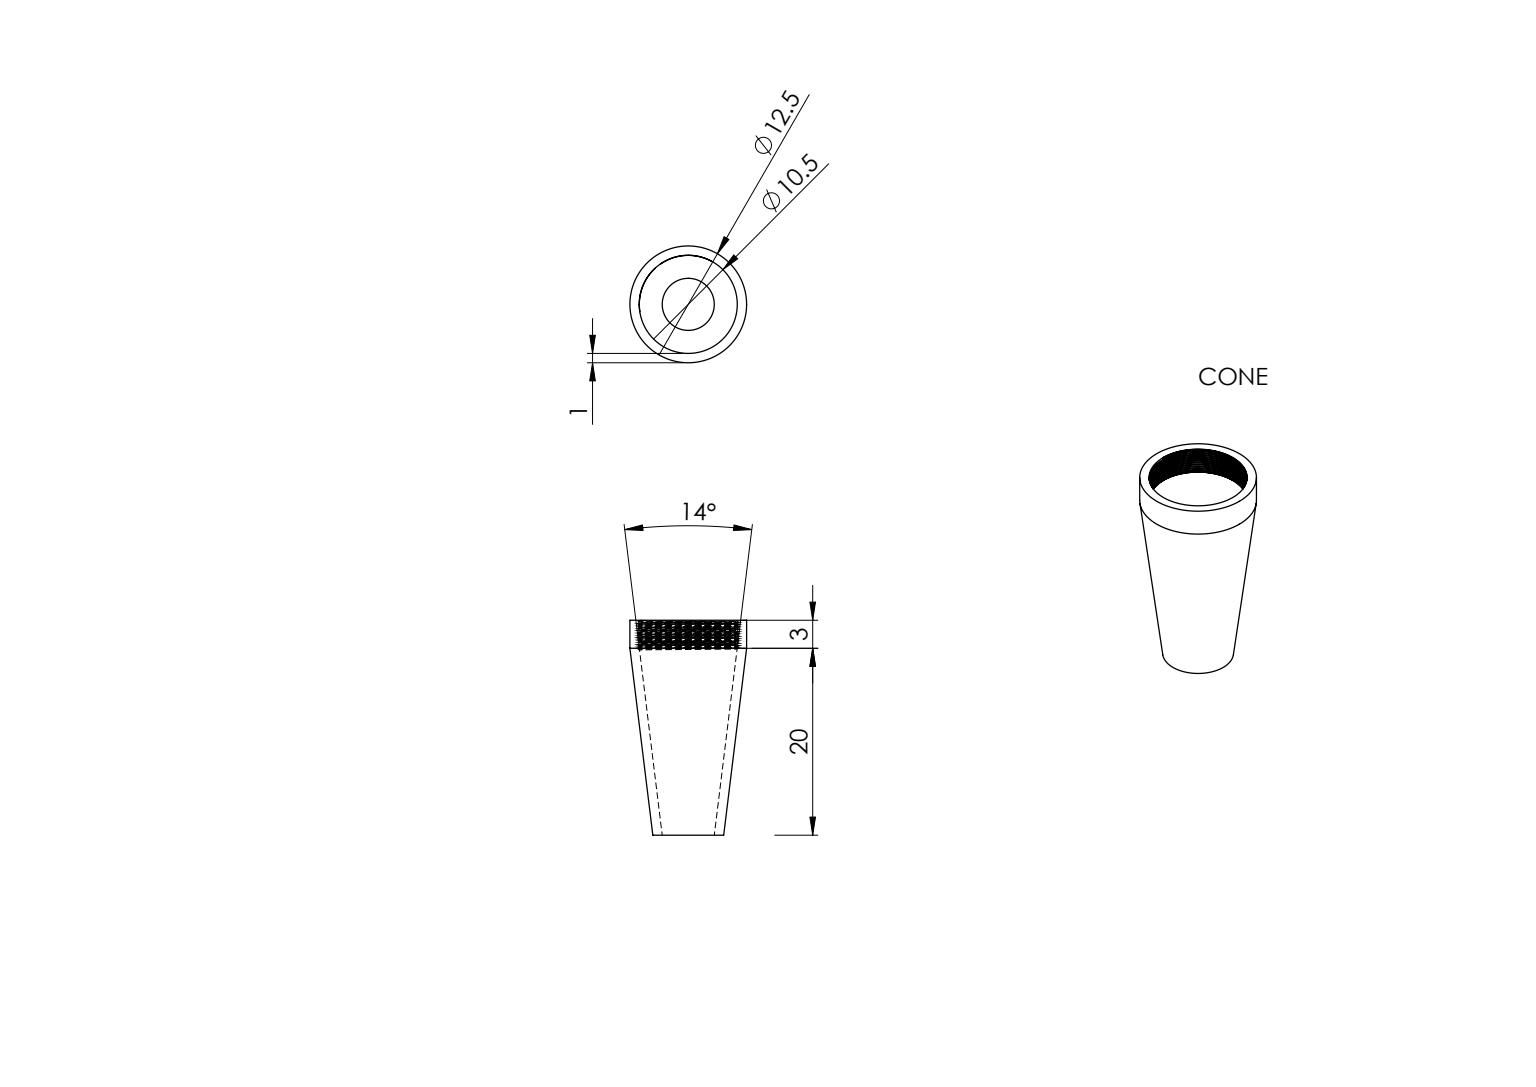
ISO-10303-21;
HEADER;
FILE_DESCRIPTION (('STEP AP214'),
    '1' );
FILE_NAME ('cone.step',
    '2026-10-27T10:49:47',
    ( '' ),
    ( '' ),
    'SwSTEP 2.0',
    'SolidWorks 2026',
    '' );
FILE_SCHEMA (( 'AUTOMOTIVE_DESIGN' ));
ENDSEC;

DATA;
#3=CARTESIAN_POINT ( 'NONE',  ( 1.113604000661152470E-15, -29.93749999999999645, 6.062177826491070398 ) ) ;
#13=CARTESIAN_POINT ( 'NONE',  ( 2.625000000000002220, -29.35416666598386826, 4.546633369868302132 ) ) ;
#14=CARTESIAN_POINT ( 'NONE',  ( 5.249999999999999112, -27.54166666598387181, -3.031088913245536975 ) ) ;
#20=CARTESIAN_POINT ( 'NONE',  ( -5.249999999999997335, -28.91666666598386826, 3.031088913245538308 ) ) ;
#27=VERTEX_POINT ( 'NONE', #2510 ) ;
#29=CARTESIAN_POINT ( 'NONE',  ( 6.429395695523604153E-16, -27.00000000000000000, 5.250000000000000000 ) ) ;
#31=CARTESIAN_POINT ( 'NONE',  ( 2.625000000000002220, -28.91666666666666785, 4.546633369868302132 ) ) ;
#34=CARTESIAN_POINT ( 'NONE',  ( -5.249999999999999112, -28.70833333265053611, -3.031088913245534755 ) ) ;
#38=CARTESIAN_POINT ( 'NONE',  ( 1.406733260263403507, -28.57366454968462577, -5.249999999999994671 ) ) ;
#39=CARTESIAN_POINT ( 'NONE',  ( 5.385316468750000141, -27.73437499965860198, -6.595110575850215044E-16 ) ) ;
#43=APPLICATION_CONTEXT ( 'automotive_design' ) ;
#46=CARTESIAN_POINT ( 'NONE',  ( 5.385316468750000141, -27.45312499965860198, -6.595110575850215044E-16 ) ) ;
#48=ORIENTED_EDGE ( 'NONE', *, *, #6878, .T. ) ;
#49=CARTESIAN_POINT ( 'NONE',  ( -5.385316468750000141, -27.32812499965860198, 0.000000000000000000 ) ) ;
#51=ORIENTED_EDGE ( 'NONE', *, *, #9169, .T. ) ;
#53=CYLINDRICAL_SURFACE ( 'NONE', #3617, 5.250000000000000000 ) ;
#58=CARTESIAN_POINT ( 'NONE',  ( 2.324088772396477476E-15, -27.49999999931720751, -5.250000000000000000 ) ) ;
#60=LINE ( 'NONE', #4208, #5677 ) ;
#63=EDGE_LOOP ( 'NONE', ( #2688, #9138, #7959, #2580 ) ) ;
#64=CARTESIAN_POINT ( 'NONE',  ( 2.161402558328724325E-14, -28.99999999931720751, -5.250000000000000000 ) ) ;
#67=ORIENTED_EDGE ( 'NONE', *, *, #7886, .F. ) ;
#68=DIRECTION ( 'NONE',  ( 0.000000000000000000, -1.000000000000000000, 0.000000000000000000 ) ) ;
#71=EDGE_LOOP ( 'NONE', ( #3557, #48, #247, #244 ) ) ;
#81=CARTESIAN_POINT ( 'NONE',  ( -3.807688866302469071E-16, -28.17187499965860553, -6.218427825808274356 ) ) ;
#85=( BOUNDED_CURVE ( )  B_SPLINE_CURVE ( 2, ( #9078, #8390, #6906, #2534, #530 ),
 .UNSPECIFIED., .F., .F. ) 
 B_SPLINE_CURVE_WITH_KNOTS ( ( 3, 2, 3 ),
 ( 0.9791666666666667407, 0.9861111111111111605, 1.000000000000000000 ),
 .UNSPECIFIED. ) 
 CURVE ( )  GEOMETRIC_REPRESENTATION_ITEM ( )  RATIONAL_B_SPLINE_CURVE ( ( 0.9330127018922192983, 0.9330127018922198534, 1.000000000000000000, 0.8660254037844387076, 1.000000000000000000 ) ) 
 REPRESENTATION_ITEM ( '' )  );
#86=ORIENTED_EDGE ( 'NONE', *, *, #5112, .F. ) ;
#87=CARTESIAN_POINT ( 'NONE',  ( -5.250000000000000000, -29.75000000000000000, 0.000000000000000000 ) ) ;
#97=EDGE_CURVE ( 'NONE', #451, #2823, #2727, .T. ) ;
#98=CARTESIAN_POINT ( 'NONE',  ( 2.161402558328724325E-14, -28.74999999931720751, -5.250000000000000000 ) ) ;
#105=VERTEX_POINT ( 'NONE', #315 ) ;
#106=CARTESIAN_POINT ( 'NONE',  ( -6.972266317189433020E-16, -27.06250000000000000, -5.250000000000000000 ) ) ;
#110=( BOUNDED_CURVE ( )  B_SPLINE_CURVE ( 2, ( #4913, #7058, #9104, #4136, #4827, #6270, #4182, #2042, #682 ),
 .UNSPECIFIED., .F., .T. ) 
 B_SPLINE_CURVE_WITH_KNOTS ( ( 3, 2, 2, 2, 3 ),
 ( 0.3541666666666666852, 0.3611111111111111049, 0.3750000000000000000, 0.3888888888888888951, 0.3958333333333333703 ),
 .UNSPECIFIED. ) 
 CURVE ( )  GEOMETRIC_REPRESENTATION_ITEM ( )  RATIONAL_B_SPLINE_CURVE ( ( 0.9330127018922194093, 0.9330127018922196314, 1.000000000000000000, 0.8660254037844387076, 1.000000000000000000, 0.8660254037844387076, 1.000000000000000000, 0.9330127018922190762, 0.9330127018922194093 ) ) 
 REPRESENTATION_ITEM ( '' )  );
#112=CARTESIAN_POINT ( 'NONE',  ( -2.033577675846918216E-14, -29.68750000000000355, 5.250000000000000888 ) ) ;
#113=CARTESIAN_POINT ( 'NONE',  ( -5.385316468750001029, -27.13020833299193413, -3.109213912904136734 ) ) ;
#119=CARTESIAN_POINT ( 'NONE',  ( -2.033577675846918216E-14, -29.87499999931720396, 5.250000000000000888 ) ) ;
#133=CARTESIAN_POINT ( 'NONE',  ( -5.385316468750000141, -28.82812499965860198, 0.000000000000000000 ) ) ;
#137=CARTESIAN_POINT ( 'NONE',  ( -2.692658234375000514, -27.61979166632526628, -4.663820869356205989 ) ) ;
#144=EDGE_CURVE ( 'NONE', #7348, #2527, #110, .T. ) ;
#160=CARTESIAN_POINT ( 'NONE',  ( 1.975475456537005874E-15, -29.62499999931719685, 5.249999999999999112 ) ) ;
#164=CARTESIAN_POINT ( 'NONE',  ( -2.625000000000000444, -27.97916666598386826, -4.546633369868303021 ) ) ;
#166=( BOUNDED_SURFACE ( )  B_SPLINE_SURFACE ( 1, 2, ( 
 ( #818, #6351, #7897, #2127, #6396, #4313, #4951, #7148, #3203, #6718, #3899, #5281, #6630, #911, #4591, #7235, #8126, #4545, #1608, #8029, #1563, #6587, #3708, #352, #8774, #6533, #1660, #1756, #258, #958, #3109, #3758, #6675, #8725, #7332, #4500, #215, #859, #1053, #7285, #3067, #3804, #3016, #5234, #5886, #5091, #4447, #167, #2357, #7377, #305, #5186, #5841, #6023, #5933, #2404, #8079, #8680, #1707, #1003, #7942, #3849, #2312, #3158, #5976, #8819, #2455, #2263, #5138, #7428, #4404, #7981, #4124, #8269, #545, #7618, #1856, #6123, #7569, #1243, #4085, #4819, #1104, #6920, #1900, #6958, #1989, #4775, #589, #3433, #1946, #3386, #1149, #4683, #3246, #6823, #6218, #8223, #2553, #7663, #8860, #9047, #5420, #6173, #4636, #5373, #7474, #7520, #2500, #399, #2692, #8952, #6772, #3992, #5323, #5519, #8364, #1285, #6070, #8177, #449, #1803, #3295, #6873, #3944, #4728, #1198, #499, #2603, #4041, #8906, #3344, #9000, #2647, #5469, #8315, #2033, #1328, #7703, #4856, #8406, #9093, #5561, #7005, #630 ),
 ( #2737, #6262, #4171, #7436, #8826, #964, #4457, #8135, #1571, #2461, #8086, #5147, #2366, #5099, #918, #7244, #1061, #3117, #868, #5196, #5286, #3811, #4510, #6636, #7294, #1010, #3073, #1667, #8038, #3905, #1713, #4552, #3768, #1618, #175, #6595, #7386, #7989, #8688, #1763, #6728, #3164, #7339, #5940, #4413, #2319, #3718, #225, #359, #6543, #3858, #5894, #3027, #8734, #2272, #4598, #5802, #8640, #5849, #6681, #265, #7949, #8782, #2411, #5242, #311, #5985, #6950, #6995, #2773, #3551, #4115, #2023, #5510, #3463, #579, #8353, #621, #750, #2861, #2724, #703, #4808, #4933, #3423, #5679, #6373, #1978, #4848, #6209, #7694, #4247, #7790, #7127, #5637, #6331, #2063, #2107, #8526, #2680, #9084, #8397, #9038, #6252, #13, #5593, #2816, #7654, #5551, #1277, #7039, #1318, #4891, #1408, #8486, #7743, #4162, #6292, #9128, #1447, #4291, #8437, #9167, #7081, #2155, #664, #1365, #4204, #3508, #4974, #7828, #5912, #4337, #7263, #4428, #797, #1687, #1544, #3641, #4527, #2335, #7172, #5215, #839, #7357 ) ),
 .UNSPECIFIED., .F., .F., .T. ) 
 B_SPLINE_SURFACE_WITH_KNOTS ( ( 2, 2 ),
 ( 3, 2, 2, 2, 2, 2, 2, 2, 2, 2, 2, 2, 2, 2, 2, 2, 2, 2, 2, 2, 2, 2, 2, 2, 2, 2, 2, 2, 2, 2, 2, 2, 2, 2, 2, 2, 2, 2, 2, 2, 2, 2, 2, 2, 2, 2, 2, 2, 2, 2, 2, 2, 2, 2, 2, 2, 2, 2, 2, 2, 2, 2, 2, 2, 2, 2, 2, 2, 2, 2, 2, 2, 3 ),
 ( 0.000000000000000000, 1.000000000000000000 ),
 ( 0.000000000000000000, 0.01388888888888888812, 0.02777777777777777624, 0.04166666666666666435, 0.05555555555555555247, 0.06944444444444444753, 0.08333333333333332871, 0.09722222222222222376, 0.1111111111111111049, 0.1250000000000000000, 0.1388888888888888951, 0.1527777777777777901, 0.1666666666666666574, 0.1805555555555555525, 0.1944444444444444475, 0.2083333333333333426, 0.2222222222222222099, 0.2361111111111111049, 0.2500000000000000000, 0.2638888888888888951, 0.2777777777777777901, 0.2916666666666666852, 0.3055555555555555802, 0.3194444444444444198, 0.3333333333333333148, 0.3472222222222222099, 0.3611111111111111049, 0.3750000000000000000, 0.3888888888888888951, 0.4027777777777777901, 0.4166666666666666852, 0.4305555555555555802, 0.4444444444444444198, 0.4583333333333333148, 0.4722222222222222099, 0.4861111111111111049, 0.5000000000000000000, 0.5138888888888888395, 0.5277777777777777901, 0.5416666666666666297, 0.5555555555555555802, 0.5694444444444444198, 0.5833333333333333703, 0.5972222222222222099, 0.6111111111111111605, 0.6250000000000000000, 0.6388888888888888395, 0.6527777777777777901, 0.6666666666666666297, 0.6805555555555555802, 0.6944444444444444198, 0.7083333333333333703, 0.7222222222222222099, 0.7361111111111111605, 0.7500000000000000000, 0.7638888888888888395, 0.7777777777777777901, 0.7916666666666666297, 0.8055555555555555802, 0.8194444444444444198, 0.8333333333333333703, 0.8472222222222222099, 0.8611111111111111605, 0.8750000000000000000, 0.8888888888888888395, 0.9027777777777777901, 0.9166666666666666297, 0.9305555555555555802, 0.9444444444444444198, 0.9583333333333333703, 0.9722222222222222099, 0.9861111111111111605, 1.000000000000000000 ),
 .UNSPECIFIED. ) 
 GEOMETRIC_REPRESENTATION_ITEM ( )  RATIONAL_B_SPLINE_SURFACE ( (
 ( 1.000000000000000000, 0.8660254037844387076, 1.000000000000000000, 0.8660254037844387076, 1.000000000000000000, 0.8660254037844387076, 1.000000000000000000, 0.8660254037844387076, 1.000000000000000000, 0.8660254037844387076, 1.000000000000000000, 0.8660254037844387076, 1.000000000000000000, 0.8660254037844387076, 1.000000000000000000, 0.8660254037844387076, 1.000000000000000000, 0.8660254037844387076, 1.000000000000000000, 0.8660254037844387076, 1.000000000000000000, 0.8660254037844387076, 1.000000000000000000, 0.8660254037844387076, 1.000000000000000000, 0.8660254037844387076, 1.000000000000000000, 0.8660254037844387076, 1.000000000000000000, 0.8660254037844387076, 1.000000000000000000, 0.8660254037844387076, 1.000000000000000000, 0.8660254037844387076, 1.000000000000000000, 0.8660254037844387076, 1.000000000000000000, 0.8660254037844387076, 1.000000000000000000, 0.8660254037844387076, 1.000000000000000000, 0.8660254037844387076, 1.000000000000000000, 0.8660254037844387076, 1.000000000000000000, 0.8660254037844387076, 1.000000000000000000, 0.8660254037844387076, 1.000000000000000000, 0.8660254037844387076, 1.000000000000000000, 0.8660254037844387076, 1.000000000000000000, 0.8660254037844387076, 1.000000000000000000, 0.8660254037844387076, 1.000000000000000000, 0.8660254037844387076, 1.000000000000000000, 0.8660254037844387076, 1.000000000000000000, 0.8660254037844387076, 1.000000000000000000, 0.8660254037844387076, 1.000000000000000000, 0.8660254037844387076, 1.000000000000000000, 0.8660254037844387076, 1.000000000000000000, 0.8660254037844387076, 1.000000000000000000, 0.8660254037844387076, 1.000000000000000000, 0.8660254037844387076, 1.000000000000000000, 0.8660254037844387076, 1.000000000000000000, 0.8660254037844387076, 1.000000000000000000, 0.8660254037844387076, 1.000000000000000000, 0.8660254037844387076, 1.000000000000000000, 0.8660254037844387076, 1.000000000000000000, 0.8660254037844387076, 1.000000000000000000, 0.8660254037844387076, 1.000000000000000000, 0.8660254037844387076, 1.000000000000000000, 0.8660254037844387076, 1.000000000000000000, 0.8660254037844387076, 1.000000000000000000, 0.8660254037844387076, 1.000000000000000000, 0.8660254037844387076, 1.000000000000000000, 0.8660254037844387076, 1.000000000000000000, 0.8660254037844387076, 1.000000000000000000, 0.8660254037844387076, 1.000000000000000000, 0.8660254037844387076, 1.000000000000000000, 0.8660254037844387076, 1.000000000000000000, 0.8660254037844387076, 1.000000000000000000, 0.8660254037844387076, 1.000000000000000000, 0.8660254037844387076, 1.000000000000000000, 0.8660254037844387076, 1.000000000000000000, 0.8660254037844387076, 1.000000000000000000, 0.8660254037844387076, 1.000000000000000000, 0.8660254037844387076, 1.000000000000000000, 0.8660254037844387076, 1.000000000000000000, 0.8660254037844387076, 1.000000000000000000, 0.8660254037844387076, 1.000000000000000000, 0.8660254037844387076, 1.000000000000000000, 0.8660254037844387076, 1.000000000000000000, 0.8660254037844387076, 1.000000000000000000, 0.8660254037844387076, 1.000000000000000000, 0.8660254037844387076, 1.000000000000000000, 0.8660254037844387076, 1.000000000000000000, 0.8660254037844387076, 1.000000000000000000, 0.8660254037844387076, 1.000000000000000000),
 ( 1.000000000000000000, 0.8660254037844387076, 1.000000000000000000, 0.8660254037844387076, 1.000000000000000000, 0.8660254037844387076, 1.000000000000000000, 0.8660254037844387076, 1.000000000000000000, 0.8660254037844387076, 1.000000000000000000, 0.8660254037844387076, 1.000000000000000000, 0.8660254037844387076, 1.000000000000000000, 0.8660254037844387076, 1.000000000000000000, 0.8660254037844387076, 1.000000000000000000, 0.8660254037844387076, 1.000000000000000000, 0.8660254037844387076, 1.000000000000000000, 0.8660254037844387076, 1.000000000000000000, 0.8660254037844387076, 1.000000000000000000, 0.8660254037844387076, 1.000000000000000000, 0.8660254037844387076, 1.000000000000000000, 0.8660254037844387076, 1.000000000000000000, 0.8660254037844387076, 1.000000000000000000, 0.8660254037844387076, 1.000000000000000000, 0.8660254037844387076, 1.000000000000000000, 0.8660254037844387076, 1.000000000000000000, 0.8660254037844387076, 1.000000000000000000, 0.8660254037844387076, 1.000000000000000000, 0.8660254037844387076, 1.000000000000000000, 0.8660254037844387076, 1.000000000000000000, 0.8660254037844387076, 1.000000000000000000, 0.8660254037844387076, 1.000000000000000000, 0.8660254037844387076, 1.000000000000000000, 0.8660254037844387076, 1.000000000000000000, 0.8660254037844387076, 1.000000000000000000, 0.8660254037844387076, 1.000000000000000000, 0.8660254037844387076, 1.000000000000000000, 0.8660254037844387076, 1.000000000000000000, 0.8660254037844387076, 1.000000000000000000, 0.8660254037844387076, 1.000000000000000000, 0.8660254037844387076, 1.000000000000000000, 0.8660254037844387076, 1.000000000000000000, 0.8660254037844387076, 1.000000000000000000, 0.8660254037844387076, 1.000000000000000000, 0.8660254037844387076, 1.000000000000000000, 0.8660254037844387076, 1.000000000000000000, 0.8660254037844387076, 1.000000000000000000, 0.8660254037844387076, 1.000000000000000000, 0.8660254037844387076, 1.000000000000000000, 0.8660254037844387076, 1.000000000000000000, 0.8660254037844387076, 1.000000000000000000, 0.8660254037844387076, 1.000000000000000000, 0.8660254037844387076, 1.000000000000000000, 0.8660254037844387076, 1.000000000000000000, 0.8660254037844387076, 1.000000000000000000, 0.8660254037844387076, 1.000000000000000000, 0.8660254037844387076, 1.000000000000000000, 0.8660254037844387076, 1.000000000000000000, 0.8660254037844387076, 1.000000000000000000, 0.8660254037844387076, 1.000000000000000000, 0.8660254037844387076, 1.000000000000000000, 0.8660254037844387076, 1.000000000000000000, 0.8660254037844387076, 1.000000000000000000, 0.8660254037844387076, 1.000000000000000000, 0.8660254037844387076, 1.000000000000000000, 0.8660254037844387076, 1.000000000000000000, 0.8660254037844387076, 1.000000000000000000, 0.8660254037844387076, 1.000000000000000000, 0.8660254037844387076, 1.000000000000000000, 0.8660254037844387076, 1.000000000000000000, 0.8660254037844387076, 1.000000000000000000, 0.8660254037844387076, 1.000000000000000000, 0.8660254037844387076, 1.000000000000000000, 0.8660254037844387076, 1.000000000000000000, 0.8660254037844387076, 1.000000000000000000, 0.8660254037844387076, 1.000000000000000000, 0.8660254037844387076, 1.000000000000000000, 0.8660254037844387076, 1.000000000000000000) ) ) 
 REPRESENTATION_ITEM ( '' )  SURFACE ( )  );
#167=CARTESIAN_POINT ( 'NONE',  ( -5.385316468749998364, -28.08854166632526628, 3.109213912904140287 ) ) ;
#170=CARTESIAN_POINT ( 'NONE',  ( 1.142306659890740623E-15, -27.26562499965860553, 6.218427825808274356 ) ) ;
#172=CARTESIAN_POINT ( 'NONE',  ( -5.249999999999997335, -29.41666666598387181, 3.031088913245538308 ) ) ;
#173=EDGE_CURVE ( 'NONE', #105, #7348, #3624, .T. ) ;
#175=CARTESIAN_POINT ( 'NONE',  ( -2.624999999999996891, -27.89583333265053255, 4.546633369868304797 ) ) ;
#180=CARTESIAN_POINT ( 'NONE',  ( 1.142306659890740623E-15, -27.76562499965860198, 6.218427825808274356 ) ) ;
#182=LINE ( 'NONE', #6689, #6964 ) ;
#184=CARTESIAN_POINT ( 'NONE',  ( 2.692658234375002735, -27.24479166632526628, 4.663820869356205101 ) ) ;
#190=AXIS2_PLACEMENT_3D ( 'NONE', #7645, #6857, #8348 ) ;
#194=ADVANCED_FACE ( 'NONE', ( #7672 ), #8416, .F. ) ;
#196=CARTESIAN_POINT ( 'NONE',  ( 7.654042494670957606E-16, -27.00000000000000000, 6.250000000000000000 ) ) ;
#198=CARTESIAN_POINT ( 'NONE',  ( 0.000000000000000000, -50.00000000000000000, 0.000000000000000000 ) ) ;
#206=ADVANCED_FACE ( 'NONE', ( #2793 ), #8063, .F. ) ;
#210=CARTESIAN_POINT ( 'NONE',  ( -5.385316468750001029, -27.88020833299193413, -3.109213912904136734 ) ) ;
#215=CARTESIAN_POINT ( 'NONE',  ( -5.385316468750000141, -27.85937499965860198, 0.000000000000000000 ) ) ;
#221=DIRECTION ( 'NONE',  ( 0.000000000000000000, -1.000000000000000000, 0.000000000000000000 ) ) ;
#225=CARTESIAN_POINT ( 'NONE',  ( -5.249999999999999112, -28.16666666598386826, 3.031088913245538308 ) ) ;
#226=CARTESIAN_POINT ( 'NONE',  ( 1.045839947578414884E-14, -27.81249999999999289, -5.249999999999999112 ) ) ;
#229=CARTESIAN_POINT ( 'NONE',  ( 5.385316468749999252, -27.93229166632526628, -3.109213912904139399 ) ) ;
#231=DIRECTION ( 'NONE',  ( 1.000000000000000000, 0.000000000000000000, -0.000000000000000000 ) ) ;
#233=CARTESIAN_POINT ( 'NONE',  ( 5.385316468750000141, -27.20312499965860198, -6.595110575850215044E-16 ) ) ;
#238=CARTESIAN_POINT ( 'NONE',  ( -5.249999999999999112, -27.47916666666666430, 3.031088913245538308 ) ) ;
#241=DIRECTION ( 'NONE',  ( 0.000000000000000000, -1.000000000000000000, 0.000000000000000000 ) ) ;
#244=ORIENTED_EDGE ( 'NONE', *, *, #7027, .F. ) ;
#247=ORIENTED_EDGE ( 'NONE', *, *, #6707, .T. ) ;
#249=CARTESIAN_POINT ( 'NONE',  ( 0.000000000000000000, -27.00000000000000000, -5.250000000000000000 ) ) ;
#250=CARTESIAN_POINT ( 'NONE',  ( -2.692658234375000514, -28.15104166632526628, -4.663820869356205989 ) ) ;
#252=CARTESIAN_POINT ( 'NONE',  ( 2.625000000000002220, -29.35416666598386826, 4.546633369868302132 ) ) ;
#253=CARTESIAN_POINT ( 'NONE',  ( -2.692658234375000514, -27.90104166632526628, -4.663820869356205989 ) ) ;
#255=CARTESIAN_POINT ( 'NONE',  ( -6.438524027057392246E-16, -29.87813065659485190, 5.257453848358681014 ) ) ;
#258=CARTESIAN_POINT ( 'NONE',  ( 2.692658234374998738, -27.69270833299193768, -4.663820869356206877 ) ) ;
#263=DIRECTION ( 'NONE',  ( 0.000000000000000000, 0.000000000000000000, -1.000000000000000000 ) ) ;
#265=CARTESIAN_POINT ( 'NONE',  ( -5.250000000000000000, -28.43749999931720396, 0.000000000000000000 ) ) ;
#269=DIRECTION ( 'NONE',  ( -1.492469013153037857E-17, 0.9925461516413219831, 0.1218693434051477398 ) ) ;
#271=CARTESIAN_POINT ( 'NONE',  ( -2.692658234374996518, -28.03645833299193413, 4.663820869356208654 ) ) ;
#275=CARTESIAN_POINT ( 'NONE',  ( -5.385316468750001029, -28.34895833299193058, -3.109213912904136734 ) ) ;
#279=VECTOR ( 'NONE', #5592, 1000.000000000000000 ) ;
#281=ORIENTED_EDGE ( 'NONE', *, *, #4233, .T. ) ;
#291=ORIENTED_EDGE ( 'NONE', *, *, #7027, .T. ) ;
#300=CARTESIAN_POINT ( 'NONE',  ( -5.385316468750001029, -27.88020833299193413, -3.109213912904136734 ) ) ;
#301=VERTEX_POINT ( 'NONE', #7582 ) ;
#305=CARTESIAN_POINT ( 'NONE',  ( -2.692658234375000514, -28.15104166632526628, -4.663820869356205989 ) ) ;
#307=ORIENTED_EDGE ( 'NONE', *, *, #1659, .F. ) ;
#310=CARTESIAN_POINT ( 'NONE',  ( 1.975475456537005874E-15, -27.43750000000000000, 5.249999999999999112 ) ) ;
#311=CARTESIAN_POINT ( 'NONE',  ( 5.250000000000000000, -28.54166666598386826, -3.031088913245536531 ) ) ;
#313=EDGE_CURVE ( 'NONE', #7348, #2202, #1209, .T. ) ;
#314=CARTESIAN_POINT ( 'NONE',  ( 0.000000000000000000, -27.00000000000000000, 0.000000000000000000 ) ) ;
#315=CARTESIAN_POINT ( 'NONE',  ( 1.975475456537005874E-15, -28.12499999931720041, 5.249999999999999112 ) ) ;
#317=CARTESIAN_POINT ( 'NONE',  ( 5.385316468750000141, -28.20312499965860198, -6.595110575850215044E-16 ) ) ;
#319=CARTESIAN_POINT ( 'NONE',  ( -2.624999999999996891, -28.45833333333333215, 4.546633369868304797 ) ) ;
#321=CARTESIAN_POINT ( 'NONE',  ( 1.142306659890740623E-15, -28.01562499965860553, 6.218427825808274356 ) ) ;
#323=ORIENTED_EDGE ( 'NONE', *, *, #5988, .F. ) ;
#334=CARTESIAN_POINT ( 'NONE',  ( -5.385316468750000141, -30.09374999965860198, 0.000000000000000000 ) ) ;
#340=VECTOR ( 'NONE', #6184, 1000.000000000000000 ) ;
#342=CARTESIAN_POINT ( 'NONE',  ( -2.692658234374996518, -29.31770833299193413, 4.663820869356208654 ) ) ;
#347=CARTESIAN_POINT ( 'NONE',  ( 5.385316468750001029, -28.75520833299193413, 3.109213912904135846 ) ) ;
#348=EDGE_LOOP ( 'NONE', ( #4332, #2732, #6898, #1040, #4602, #5151, #8448, #421, #7230, #5370, #7405, #1528, #896, #3291, #5973, #7049, #8359, #4121, #7939, #1869, #4062, #7510, #7908, #3823, #5397, #1583, #3967 ) ) ;
#352=CARTESIAN_POINT ( 'NONE',  ( -5.385316468749998364, -27.58854166632526983, 3.109213912904140287 ) ) ;
#354=CARTESIAN_POINT ( 'NONE',  ( -2.692658234374996518, -28.03645833299193413, 4.663820869356208654 ) ) ;
#359=CARTESIAN_POINT ( 'NONE',  ( -5.250000000000000000, -28.18749999931720396, 0.000000000000000000 ) ) ;
#360=CARTESIAN_POINT ( 'NONE',  ( -2.625000000000000444, -28.47916666598386826, -4.546633369868303021 ) ) ;
#365=CARTESIAN_POINT ( 'NONE',  ( 2.692658234374998738, -29.91145833299193413, -4.663820869356206877 ) ) ;
#368=CARTESIAN_POINT ( 'NONE',  ( -5.385316468750000141, -27.09374999965859843, 0.000000000000000000 ) ) ;
#370=CARTESIAN_POINT ( 'NONE',  ( 2.692658234375002735, -27.99479166632526628, 4.663820869356205101 ) ) ;
#374=CARTESIAN_POINT ( 'NONE',  ( 1.406733260263393293, -27.07366454968463287, -5.250000000000000000 ) ) ;
#377=FACE_OUTER_BOUND ( 'NONE', #6458, .T. ) ;
#381=CARTESIAN_POINT ( 'NONE',  ( -6.972266317189433020E-16, -27.56249999999999645, -5.249999999999999112 ) ) ;
#387=( BOUNDED_CURVE ( )  B_SPLINE_CURVE ( 2, ( #1018, #3037, #319, #6552, #8833, #8095, #5950, #3912, #3776 ),
 .UNSPECIFIED., .F., .F. ) 
 B_SPLINE_CURVE_WITH_KNOTS ( ( 3, 2, 2, 2, 3 ),
 ( 0.4791666666666666852, 0.4861111111111111049, 0.5000000000000000000, 0.5138888888888888395, 0.5208333333333333703 ),
 .UNSPECIFIED. ) 
 CURVE ( )  GEOMETRIC_REPRESENTATION_ITEM ( )  RATIONAL_B_SPLINE_CURVE ( ( 0.9330127018922194093, 0.9330127018922196314, 1.000000000000000000, 0.8660254037844387076, 1.000000000000000000, 0.8660254037844387076, 1.000000000000000000, 0.9330127018922187432, 0.9330127018922192983 ) ) 
 REPRESENTATION_ITEM ( '' )  );
#389=FACE_OUTER_BOUND ( 'NONE', #1082, .T. ) ;
#390=CARTESIAN_POINT ( 'NONE',  ( 2.692658234374998738, -29.44270833299193413, -4.663820869356206877 ) ) ;
#394=CARTESIAN_POINT ( 'NONE',  ( 2.692658234375002735, -29.77604166632526983, 4.663820869356205101 ) ) ;
#396=EDGE_LOOP ( 'NONE', ( #8293, #5107, #8604, #2518 ) ) ;
#399=CARTESIAN_POINT ( 'NONE',  ( -5.385316468750001029, -29.38020833299193413, -3.109213912904136734 ) ) ;
#401=CARTESIAN_POINT ( 'NONE',  ( 2.692658234375002735, -28.24479166632526628, 4.663820869356205101 ) ) ;
#410=CARTESIAN_POINT ( 'NONE',  ( -2.692658234375000514, -29.61979166632526983, -4.663820869356205989 ) ) ;
#413=CARTESIAN_POINT ( 'NONE',  ( 2.692658234374998738, -28.41145833299193413, -4.663820869356206877 ) ) ;
#415=ORIENTED_EDGE ( 'NONE', *, *, #2354, .T. ) ;
#421=ORIENTED_EDGE ( 'NONE', *, *, #2572, .T. ) ;
#422=CARTESIAN_POINT ( 'NONE',  ( 5.250000000000000000, -28.35416666666666785, -3.031088913245536531 ) ) ;
#427=LINE ( 'NONE', #7410, #8373 ) ;
#429=CARTESIAN_POINT ( 'NONE',  ( -5.249999999999999112, -29.20833333265053611, -3.031088913245534755 ) ) ;
#435=EDGE_CURVE ( 'NONE', #6343, #8584, #1529, .T. ) ;
#437=ORIENTED_EDGE ( 'NONE', *, *, #2736, .F. ) ;
#439=CARTESIAN_POINT ( 'NONE',  ( 5.385316468750000141, -28.23437499965860198, -6.595110575850215044E-16 ) ) ;
#442=CARTESIAN_POINT ( 'NONE',  ( 2.692658234374998738, -29.44270833299193413, -4.663820869356206877 ) ) ;
#445=ORIENTED_EDGE ( 'NONE', *, *, #3049, .T. ) ;
#449=CARTESIAN_POINT ( 'NONE',  ( -5.385316468750000141, -29.60937499965859843, 0.000000000000000000 ) ) ;
#451=VERTEX_POINT ( 'NONE', #8588 ) ;
#452=CARTESIAN_POINT ( 'NONE',  ( -5.385316468750001029, -28.09895833299192702, -3.109213912904136734 ) ) ;
#457=CARTESIAN_POINT ( 'NONE',  ( 1.975475456537005874E-15, -27.18750000000000000, 5.249999999999999112 ) ) ;
#458=CARTESIAN_POINT ( 'NONE',  ( 1.975475456537005874E-15, -27.43750000000000000, 5.250000000000000000 ) ) ;
#462=CARTESIAN_POINT ( 'NONE',  ( -2.692658234375000514, -29.86979166632526983, -4.663820869356205989 ) ) ;
#465=CARTESIAN_POINT ( 'NONE',  ( 5.385316468750001029, -28.97395833299193413, 3.109213912904135846 ) ) ;
#471=( BOUNDED_CURVE ( )  B_SPLINE_CURVE ( 2, ( #670, #9175, #628, #9136, #1283, #3603, #5600, #2161, #6260 ),
 .UNSPECIFIED., .F., .T. ) 
 B_SPLINE_CURVE_WITH_KNOTS ( ( 3, 2, 2, 2, 3 ),
 ( 0.6875000000000000000, 0.6944444444444444198, 0.7083333333333333703, 0.7222222222222222099, 0.7291666666666667407 ),
 .UNSPECIFIED. ) 
 CURVE ( )  GEOMETRIC_REPRESENTATION_ITEM ( )  RATIONAL_B_SPLINE_CURVE ( ( 0.9330127018922194093, 0.9330127018922194093, 1.000000000000000000, 0.8660254037844387076, 1.000000000000000000, 0.8660254037844387076, 1.000000000000000000, 0.9330127018922187432, 0.9330127018922192983 ) ) 
 REPRESENTATION_ITEM ( '' )  );
#473=( LENGTH_UNIT ( ) NAMED_UNIT ( * ) SI_UNIT ( .MILLI., .METRE. ) );
#474=CARTESIAN_POINT ( 'NONE',  ( 2.625000000000002220, -28.16666666666666785, 4.546633369868302132 ) ) ;
#480=CARTESIAN_POINT ( 'NONE',  ( -2.624999999999996891, -29.14583333265053611, 4.546633369868304797 ) ) ;
#481=ADVANCED_FACE ( 'NONE', ( #820 ), #7102, .F. ) ;
#486=ADVANCED_FACE ( 'NONE', ( #726 ), #5094, .F. ) ;
#487=PLANE ( 'NONE',  #4222 ) ;
#488=CARTESIAN_POINT ( 'NONE',  ( -2.692658234374996518, -28.56770833299193413, 4.663820869356208654 ) ) ;
#489=CARTESIAN_POINT ( 'NONE',  ( -5.385316468750000141, -29.60937499965859843, 0.000000000000000000 ) ) ;
#491=CARTESIAN_POINT ( 'NONE',  ( 2.692658234375002735, -28.77604166632526628, 4.663820869356205101 ) ) ;
#499=CARTESIAN_POINT ( 'NONE',  ( 5.385316468750001029, -29.75520833299193413, 3.109213912904135846 ) ) ;
#503=CARTESIAN_POINT ( 'NONE',  ( -2.692658234374996518, -28.53645833299193413, 4.663820869356208654 ) ) ;
#506=AXIS2_PLACEMENT_3D ( 'NONE', #1402, #9122, #6460 ) ;
#511=DIRECTION ( 'NONE',  ( 0.000000000000000000, 0.000000000000000000, -1.000000000000000000 ) ) ;
#512=CARTESIAN_POINT ( 'NONE',  ( -2.692658234375000514, -29.36979166632526983, -4.663820869356205989 ) ) ;
#516=CARTESIAN_POINT ( 'NONE',  ( -2.692658234374996518, -29.53645833299193413, 4.663820869356208654 ) ) ;
#520=FACE_OUTER_BOUND ( 'NONE', #7413, .T. ) ;
#523=ORIENTED_EDGE ( 'NONE', *, *, #4456, .T. ) ;
#524=CARTESIAN_POINT ( 'NONE',  ( 5.250000000000000888, -28.39583333333333215, 3.031088913245532979 ) ) ;
#530=CARTESIAN_POINT ( 'NONE',  ( -5.250000000000000000, -30.00000000000000000, 0.000000000000000000 ) ) ;
#535=CARTESIAN_POINT ( 'NONE',  ( -5.385316468749998364, -29.08854166632526983, 3.109213912904140287 ) ) ;
#536=CARTESIAN_POINT ( 'NONE',  ( 2.692658234374998738, -29.69270833299193413, -4.663820869356206877 ) ) ;
#538=CARTESIAN_POINT ( 'NONE',  ( 5.385316468750000141, -28.98437499965859843, -6.595110575850215044E-16 ) ) ;
#545=CARTESIAN_POINT ( 'NONE',  ( -2.692658234375000514, -28.65104166632526628, -4.663820869356205989 ) ) ;
#546=EDGE_CURVE ( 'NONE', #27, #4503, #1592, .T. ) ;
#548=CARTESIAN_POINT ( 'NONE',  ( 5.385316468750000141, -28.20312499965860198, -6.595110575850215044E-16 ) ) ;
#551=DIRECTION ( 'NONE',  ( 0.000000000000000000, -1.000000000000000000, 0.000000000000000000 ) ) ;
#558=CARTESIAN_POINT ( 'NONE',  ( -5.385316468750001029, -29.34895833299193413, -3.109213912904136734 ) ) ;
#561=CARTESIAN_POINT ( 'NONE',  ( -2.692658234374996518, -27.31770833299193413, 4.663820869356208654 ) ) ;
#563=DIRECTION ( 'NONE',  ( 0.000000000000000000, 0.000000000000000000, -1.000000000000000000 ) ) ;
#567=CARTESIAN_POINT ( 'NONE',  ( 2.624999999999998668, -28.33333333333333215, -4.546633369868303021 ) ) ;
#570=CARTESIAN_POINT ( 'NONE',  ( 5.250000000000000000, -28.12500000000000000, -6.429395695523604153E-16 ) ) ;
#577=CARTESIAN_POINT ( 'NONE',  ( -5.249999999999997335, -29.22916666666666785, 3.031088913245538308 ) ) ;
#579=CARTESIAN_POINT ( 'NONE',  ( -3.712013335537174572E-16, -28.74999999931720396, -6.062177826491070398 ) ) ;
#580=CARTESIAN_POINT ( 'NONE',  ( -2.692658234375000514, -29.65104166632526983, -4.663820869356205989 ) ) ;
#585=EDGE_LOOP ( 'NONE', ( #8972, #8285, #6547 ) ) ;
#586=AXIS2_PLACEMENT_3D ( 'NONE', #3012, #4443, #8023 ) ;
#589=CARTESIAN_POINT ( 'NONE',  ( 2.692658234374998738, -28.94270833299193413, -4.663820869356206877 ) ) ;
#592=CARTESIAN_POINT ( 'NONE',  ( 1.142306659890740623E-15, -29.01562499965860198, 6.218427825808274356 ) ) ;
#595=CARTESIAN_POINT ( 'NONE',  ( -5.317658234375000070, -27.03906249982929921, 0.000000000000000000 ) ) ;
#597=FACE_OUTER_BOUND ( 'NONE', #7205, .T. ) ;
#599=DIRECTION ( 'NONE',  ( -0.000000000000000000, 1.000000000000000000, -0.000000000000000000 ) ) ;
#601=CARTESIAN_POINT ( 'NONE',  ( -2.625000000000000444, -28.72916666598386826, -4.546633369868303021 ) ) ;
#604=CARTESIAN_POINT ( 'NONE',  ( -3.807688866302469071E-16, -29.39062499965860198, -6.218427825808274356 ) ) ;
#607=CIRCLE ( 'NONE', #1956, 2.786798956483056422 ) ;
#610=VERTEX_POINT ( 'NONE', #1167 ) ;
#611=CARTESIAN_POINT ( 'NONE',  ( -3.712013335537174572E-16, -27.81250000000000000, -6.062177826491070398 ) ) ;
#621=CARTESIAN_POINT ( 'NONE',  ( 5.250000000000000000, -28.79166666598386826, -3.031088913245536531 ) ) ;
#628=CARTESIAN_POINT ( 'NONE',  ( 2.624999999999998668, -29.08333333333333215, -4.546633369868303021 ) ) ;
#630=CARTESIAN_POINT ( 'NONE',  ( -5.385316468750000141, -30.10937499965859843, 0.000000000000000000 ) ) ;
#632=CARTESIAN_POINT ( 'NONE',  ( 5.385316468749999252, -29.43229166632526983, -3.109213912904138954 ) ) ;
#635=CARTESIAN_POINT ( 'NONE',  ( 1.975475456537005874E-15, -28.68749999999999645, 5.249999999999999112 ) ) ;
#644=CARTESIAN_POINT ( 'NONE',  ( 5.385316468750000141, -29.95312499965859843, -6.595110575850215044E-16 ) ) ;
#645=EDGE_CURVE ( 'NONE', #5282, #1598, #1067, .T. ) ;
#648=LINE ( 'NONE', #6317, #9109 ) ;
#653=ORIENTED_EDGE ( 'NONE', *, *, #4489, .T. ) ;
#655=CARTESIAN_POINT ( 'NONE',  ( 5.250000000000000000, -29.37500000000000000, -6.429395695523604153E-16 ) ) ;
#660=CARTESIAN_POINT ( 'NONE',  ( 2.161402558328724325E-14, -29.31250000000000000, -5.250000000000000000 ) ) ;
#663=CARTESIAN_POINT ( 'NONE',  ( -5.250000000000000000, -29.25000000000000000, 0.000000000000000000 ) ) ;
#664=CARTESIAN_POINT ( 'NONE',  ( 5.250000000000000000, -29.79166666598387181, -3.031088913245536531 ) ) ;
#665=CARTESIAN_POINT ( 'NONE',  ( 0.000000000000000000, -27.00000000000000000, -5.250000000000000000 ) ) ;
#670=CARTESIAN_POINT ( 'NONE',  ( -6.972266317189433020E-16, -29.06249999999999645, -5.250000000000000000 ) ) ;
#674=CARTESIAN_POINT ( 'NONE',  ( 5.385316468750001029, -29.22395833299193413, 3.109213912904134958 ) ) ;
#679=FACE_OUTER_BOUND ( 'NONE', #5811, .T. ) ;
#682=CARTESIAN_POINT ( 'NONE',  ( -9.180150650966086169E-15, -28.37499999931720041, 5.250000000000000000 ) ) ;
#685=( BOUNDED_CURVE ( )  B_SPLINE_CURVE ( 2, ( #2269, #6592, #5982, #172, #7986, #7947, #4410, #865, #3715 ),
 .UNSPECIFIED., .F., .F. ) 
 B_SPLINE_CURVE_WITH_KNOTS ( ( 3, 2, 2, 2, 3 ),
 ( 0.7291666666666667407, 0.7361111111111111605, 0.7500000000000000000, 0.7638888888888888395, 0.7708333333333333703 ),
 .UNSPECIFIED. ) 
 CURVE ( )  GEOMETRIC_REPRESENTATION_ITEM ( )  RATIONAL_B_SPLINE_CURVE ( ( 0.9330127018922192983, 0.9330127018922198534, 1.000000000000000000, 0.8660254037844387076, 1.000000000000000000, 0.8660254037844387076, 1.000000000000000000, 0.9330127018922187432, 0.9330127018922192983 ) ) 
 REPRESENTATION_ITEM ( '' )  );
#687=CARTESIAN_POINT ( 'NONE',  ( -2.692658234375000514, -29.61979166632526983, -4.663820869356205989 ) ) ;
#694=CARTESIAN_POINT ( 'NONE',  ( 5.250000000000000888, -29.39583333333332860, 3.031088913245532979 ) ) ;
#703=CARTESIAN_POINT ( 'NONE',  ( 1.113604000661152470E-15, -28.87499999931720396, 6.062177826491070398 ) ) ;
#706=CARTESIAN_POINT ( 'NONE',  ( -2.692658234374996518, -30.06770833299193413, 4.663820869356208654 ) ) ;
#713=ADVANCED_FACE ( 'NONE', ( #520 ), #7635, .F. ) ;
#715=ORIENTED_EDGE ( 'NONE', *, *, #4351, .T. ) ;
#716=CARTESIAN_POINT ( 'NONE',  ( -3.807688866302469071E-16, -29.89062499965859843, -6.218427825808274356 ) ) ;
#722=DIRECTION ( 'NONE',  ( 0.000000000000000000, 0.000000000000000000, -1.000000000000000000 ) ) ;
#726=FACE_OUTER_BOUND ( 'NONE', #1560, .T. ) ;
#730=CARTESIAN_POINT ( 'NONE',  ( -5.385316468750001029, -28.38020833299193058, -3.109213912904136734 ) ) ;
#737=CARTESIAN_POINT ( 'NONE',  ( -5.250000000000000000, -29.25000000000000000, 0.000000000000000000 ) ) ;
#739=CARTESIAN_POINT ( 'NONE',  ( -1.406733260263393070, -27.30133545031536357, -5.250000000000000888 ) ) ;
#743=EDGE_LOOP ( 'NONE', ( #7927, #7894 ) ) ;
#750=CARTESIAN_POINT ( 'NONE',  ( 5.250000000000000000, -28.81249999931720396, -6.429395695523604153E-16 ) ) ;
#751=CARTESIAN_POINT ( 'NONE',  ( 5.250000000000000000, -27.56249999931720396, -6.429395695523604153E-16 ) ) ;
#757=EDGE_LOOP ( 'NONE', ( #8210, #7399, #8601, #6496 ) ) ;
#759=CARTESIAN_POINT ( 'NONE',  ( -1.406733260263394625, -27.55133545031536713, -5.250000000000000000 ) ) ;
#761=EDGE_CURVE ( 'NONE', #7091, #2823, #648, .T. ) ;
#764=ORIENTED_EDGE ( 'NONE', *, *, #4966, .T. ) ;
#765=CARTESIAN_POINT ( 'NONE',  ( 5.385316468750000141, -29.70312499965859843, -6.595110575850215044E-16 ) ) ;
#767=CARTESIAN_POINT ( 'NONE',  ( 6.429395695523604153E-16, -27.00000000000000000, 5.250000000000000000 ) ) ;
#770=CARTESIAN_POINT ( 'NONE',  ( -6.972266317189433020E-16, -29.06249999999999645, -5.250000000000000000 ) ) ;
#771=CARTESIAN_POINT ( 'NONE',  ( 6.429395695523604153E-16, -27.00000000000000000, 5.250000000000000000 ) ) ;
#772=CARTESIAN_POINT ( 'NONE',  ( 5.250000000000000888, -27.33333333265053611, 3.031088913245533423 ) ) ;
#778=CARTESIAN_POINT ( 'NONE',  ( -2.692658234375000514, -27.65104166632526628, -4.663820869356205989 ) ) ;
#785=AXIS2_PLACEMENT_3D ( 'NONE', #1263, #6935, #563 ) ;
#786=CARTESIAN_POINT ( 'NONE',  ( 2.692658234375002735, -27.49479166632526628, 4.663820869356205101 ) ) ;
#788=ORIENTED_EDGE ( 'NONE', *, *, #7385, .F. ) ;
#797=CARTESIAN_POINT ( 'NONE',  ( -3.712013335537174572E-16, -29.99999999931720041, -6.062177826491070398 ) ) ;
#800=CARTESIAN_POINT ( 'NONE',  ( -5.250000000000000000, -27.75000000000000000, 0.000000000000000000 ) ) ;
#807=EDGE_LOOP ( 'NONE', ( #1458, #4944, #5003, #5759 ) ) ;
#809=CARTESIAN_POINT ( 'NONE',  ( 5.249999999999999112, -29.60416666666666785, -3.031088913245536975 ) ) ;
#812=CARTESIAN_POINT ( 'NONE',  ( 5.250000000000000888, -29.33333333265053611, 3.031088913245533423 ) ) ;
#814=EDGE_CURVE ( 'NONE', #4395, #3226, #6461, .T. ) ;
#818=CARTESIAN_POINT ( 'NONE',  ( -5.385316468750000141, -27.10937499965860198, 0.000000000000000000 ) ) ;
#820=FACE_OUTER_BOUND ( 'NONE', #3345, .T. ) ;
#821=CARTESIAN_POINT ( 'NONE',  ( 2.692658234374998738, -27.16145833299193413, -4.663820869356206877 ) ) ;
#823=CARTESIAN_POINT ( 'NONE',  ( 0.000000000000000000, -27.00000000000000000, 0.000000000000000000 ) ) ;
#824=CARTESIAN_POINT ( 'NONE',  ( 2.692658234375002735, -28.52604166632526628, 4.663820869356205101 ) ) ;
#829=CARTESIAN_POINT ( 'NONE',  ( 2.624999999999998668, -29.02083333265053611, -4.546633369868303021 ) ) ;
#830=EDGE_LOOP ( 'NONE', ( #2328, #67 ) ) ;
#831=CARTESIAN_POINT ( 'NONE',  ( 2.625000000000002220, -29.66666666666666785, 4.546633369868302132 ) ) ;
#839=CARTESIAN_POINT ( 'NONE',  ( -5.249999999999999112, -30.16666666598386470, 3.031088913245538308 ) ) ;
#841=LINE ( 'NONE', #941, #8467 ) ;
#842=CARTESIAN_POINT ( 'NONE',  ( -2.624999999999996891, -28.20833333333333215, 4.546633369868304797 ) ) ;
#843=CARTESIAN_POINT ( 'NONE',  ( 0.000000000000000000, -29.87813065659485190, -5.257453848358681014 ) ) ;
#846=CARTESIAN_POINT ( 'NONE',  ( 5.250000000000000888, -27.14583333333332860, 3.031088913245533423 ) ) ;
#851=EDGE_CURVE ( 'NONE', #8796, #3220, #8383, .T. ) ;
#854=CARTESIAN_POINT ( 'NONE',  ( 5.385316468749999252, -27.21354166632526628, -3.109213912904138954 ) ) ;
#857=CARTESIAN_POINT ( 'NONE',  ( 5.249999999999999112, -29.85416666666666785, -3.031088913245536975 ) ) ;
#859=CARTESIAN_POINT ( 'NONE',  ( -5.385316468750001029, -27.88020833299193413, -3.109213912904136734 ) ) ;
#860=UNCERTAINTY_MEASURE_WITH_UNIT (LENGTH_MEASURE( 1.000000000000000082E-05 ), #473, 'distance_accuracy_value', 'NONE');
#863=CARTESIAN_POINT ( 'NONE',  ( 5.385316468749999252, -27.18229166632526628, -3.109213912904138954 ) ) ;
#865=CARTESIAN_POINT ( 'NONE',  ( -1.406733260263384411, -29.48883544963257464, -5.250000000000006217 ) ) ;
#868=CARTESIAN_POINT ( 'NONE',  ( 5.250000000000000000, -27.56249999931720396, -6.429395695523604153E-16 ) ) ;
#869=CARTESIAN_POINT ( 'NONE',  ( 5.250000000000000888, -27.64583333333333570, 3.031088913245533423 ) ) ;
#876=CARTESIAN_POINT ( 'NONE',  ( 2.692658234374998738, -27.91145833299193413, -4.663820869356206877 ) ) ;
#888=AXIS2_PLACEMENT_3D ( 'NONE', #4026, #9081, #6861 ) ;
#889=CARTESIAN_POINT ( 'NONE',  ( -2.625000000000000444, -27.04166666666666430, -4.546633369868303021 ) ) ;
#896=ORIENTED_EDGE ( 'NONE', *, *, #7076, .T. ) ;
#904=CARTESIAN_POINT ( 'NONE',  ( -5.385316468750000141, -27.85937499965860198, 0.000000000000000000 ) ) ;
#911=CARTESIAN_POINT ( 'NONE',  ( -5.385316468750001029, -27.38020833299193768, -3.109213912904136734 ) ) ;
#913=DIRECTION ( 'NONE',  ( 0.000000000000000000, 0.000000000000000000, -1.000000000000000000 ) ) ;
#914=CARTESIAN_POINT ( 'NONE',  ( -5.385316468749998364, -27.55729166632526628, 3.109213912904140287 ) ) ;
#916=CARTESIAN_POINT ( 'NONE',  ( 1.975475456537005874E-15, -27.37499999931720041, 5.250000000000000000 ) ) ;
#918=CARTESIAN_POINT ( 'NONE',  ( -2.625000000000000444, -27.47916666598386826, -4.546633369868303021 ) ) ;
#923=CARTESIAN_POINT ( 'NONE',  ( -2.692658234375000514, -28.11979166632526628, -4.663820869356205989 ) ) ;
#924=EDGE_CURVE ( 'NONE', #8014, #8128, #5623, .T. ) ;
#927=ORIENTED_EDGE ( 'NONE', *, *, #5310, .F. ) ;
#928=CARTESIAN_POINT ( 'NONE',  ( -2.624999999999996891, -27.20833333333333570, 4.546633369868304797 ) ) ;
#938=CARTESIAN_POINT ( 'NONE',  ( 5.250000000000000888, -27.14583333333333570, 3.031088913245532979 ) ) ;
#941=CARTESIAN_POINT ( 'NONE',  ( 6.429395695523604153E-16, -27.00000000000000000, 5.250000000000000000 ) ) ;
#942=CARTESIAN_POINT ( 'NONE',  ( -5.250000000000000000, -28.25000000000000000, 0.000000000000000000 ) ) ;
#946=VERTEX_POINT ( 'NONE', #226 ) ;
#949=ORIENTED_EDGE ( 'NONE', *, *, #4125, .F. ) ;
#951=CARTESIAN_POINT ( 'NONE',  ( -5.385316468750001029, -27.38020833299193058, -3.109213912904136734 ) ) ;
#958=CARTESIAN_POINT ( 'NONE',  ( 5.385316468749999252, -27.71354166632526272, -3.109213912904139399 ) ) ;
#961=CARTESIAN_POINT ( 'NONE',  ( -2.692658234374996518, -27.53645833299193413, 4.663820869356208654 ) ) ;
#964=CARTESIAN_POINT ( 'NONE',  ( 5.250000000000000000, -27.29166666598386826, -3.031088913245536531 ) ) ;
#965=CARTESIAN_POINT ( 'NONE',  ( 1.975475456537005874E-15, -27.62499999931720041, 5.250000000000000000 ) ) ;
#967=CARTESIAN_POINT ( 'NONE',  ( -2.033577675846918216E-14, -29.87499999931720396, 5.250000000000000888 ) ) ;
#970=CARTESIAN_POINT ( 'NONE',  ( 2.692658234375002735, -28.24479166632526628, 4.663820869356205101 ) ) ;
#971=ADVANCED_FACE ( 'NONE', ( #8322 ), #8915, .F. ) ;
#975=CARTESIAN_POINT ( 'NONE',  ( 2.692658234374998738, -28.91145833299193413, -4.663820869356206877 ) ) ;
#982=( BOUNDED_CURVE ( )  B_SPLINE_CURVE ( 2, ( #6188, #1260, #4831, #7587, #2619, #8921, #5436, #6273, #2006 ),
 .UNSPECIFIED., .F., .F. ) 
 B_SPLINE_CURVE_WITH_KNOTS ( ( 3, 2, 2, 2, 3 ),
 ( 0.3125000000000000000, 0.3194444444444444198, 0.3333333333333333148, 0.3472222222222222099, 0.3541666666666666852 ),
 .UNSPECIFIED. ) 
 CURVE ( )  GEOMETRIC_REPRESENTATION_ITEM ( )  RATIONAL_B_SPLINE_CURVE ( ( 0.9330127018922194093, 0.9330127018922194093, 1.000000000000000000, 0.8660254037844387076, 1.000000000000000000, 0.8660254037844387076, 1.000000000000000000, 0.9330127018922190762, 0.9330127018922194093 ) ) 
 REPRESENTATION_ITEM ( '' )  );
#985=CARTESIAN_POINT ( 'NONE',  ( -1.406733260263394625, -28.30133545031536713, -5.250000000000000000 ) ) ;
#994=CARTESIAN_POINT ( 'NONE',  ( 2.692658234374998738, -27.69270833299193768, -4.663820869356206877 ) ) ;
#996=UNCERTAINTY_MEASURE_WITH_UNIT (LENGTH_MEASURE( 1.000000000000000082E-05 ), #5266, 'distance_accuracy_value', 'NONE');
#998=CARTESIAN_POINT ( 'NONE',  ( -3.807688866302469071E-16, -27.92187499965860198, -6.218427825808274356 ) ) ;
#999=ORIENTED_EDGE ( 'NONE', *, *, #4125, .T. ) ;
#1003=CARTESIAN_POINT ( 'NONE',  ( -5.385316468749998364, -28.33854166632526628, 3.109213912904140287 ) ) ;
#1005=EDGE_LOOP ( 'NONE', ( #5857, #7682, #7845, #1554 ) ) ;
#1010=CARTESIAN_POINT ( 'NONE',  ( -5.250000000000000000, -27.70833333265053611, -3.031088913245534755 ) ) ;
#1012=DIRECTION ( 'NONE',  ( 0.000000000000000000, 0.000000000000000000, -1.000000000000000000 ) ) ;
#1013=CARTESIAN_POINT ( 'NONE',  ( 1.406733260263385521, -29.11383544963257464, 5.250000000000006217 ) ) ;
#1016=CARTESIAN_POINT ( 'NONE',  ( -5.385316468749998364, -28.05729166632526983, 3.109213912904140287 ) ) ;
#1018=CARTESIAN_POINT ( 'NONE',  ( -9.180150650966086169E-15, -28.43750000000000000, 5.250000000000000000 ) ) ;
#1020=CARTESIAN_POINT ( 'NONE',  ( -5.385316468750000141, -27.82812499965860198, 0.000000000000000000 ) ) ;
#1026=ORIENTED_EDGE ( 'NONE', *, *, #3740, .T. ) ;
#1028=CARTESIAN_POINT ( 'NONE',  ( 5.250000000000000888, -27.39583333333333215, 3.031088913245532979 ) ) ;
#1035=ORIENTED_EDGE ( 'NONE', *, *, #6208, .T. ) ;
#1040=ORIENTED_EDGE ( 'NONE', *, *, #7385, .T. ) ;
#1044=CARTESIAN_POINT ( 'NONE',  ( -5.385316468749998364, -28.33854166632526628, 3.109213912904140287 ) ) ;
#1047=CARTESIAN_POINT ( 'NONE',  ( -5.385316468749998364, -28.33854166632526628, 3.109213912904140287 ) ) ;
#1053=CARTESIAN_POINT ( 'NONE',  ( -2.692658234375000514, -27.90104166632526628, -4.663820869356205989 ) ) ;
#1058=CARTESIAN_POINT ( 'NONE',  ( -5.385316468750000141, -27.82812499965860198, 0.000000000000000000 ) ) ;
#1061=CARTESIAN_POINT ( 'NONE',  ( 2.624999999999998668, -27.52083333265053611, -4.546633369868303021 ) ) ;
#1067=( BOUNDED_CURVE ( )  B_SPLINE_CURVE ( 2, ( #2665, #1920, #5537, #4010, #2757, #7722, #6844, #3964, #1877, #5392, #1965 ),
 .UNSPECIFIED., .F., .F. ) 
 B_SPLINE_CURVE_WITH_KNOTS ( ( 3, 2, 2, 2, 2, 3 ),
 ( 0.9375000002123526910, 0.9444444444444444198, 0.9583333333333333703, 0.9722222222222222099, 0.9861111111111111605, 1.000000000000000000 ),
 .UNSPECIFIED. ) 
 CURVE ( )  GEOMETRIC_REPRESENTATION_ITEM ( )  RATIONAL_B_SPLINE_CURVE ( ( 0.9330127018922194093, 0.9330127039406097555, 1.000000000000000000, 0.8660254037844387076, 1.000000000000000000, 0.8660254037844387076, 1.000000000000000000, 0.8660254037844387076, 1.000000000000000000, 0.8660254037844387076, 1.000000000000000000 ) ) 
 REPRESENTATION_ITEM ( '' )  );
#1068=CARTESIAN_POINT ( 'NONE',  ( -2.692658234375000514, -28.36979166632526628, -4.663820869356205989 ) ) ;
#1072=CARTESIAN_POINT ( 'NONE',  ( -3.807688866302469071E-16, -27.89062499965860198, -6.218427825808274356 ) ) ;
#1074=VERTEX_POINT ( 'NONE', #457 ) ;
#1079=ORIENTED_EDGE ( 'NONE', *, *, #8052, .F. ) ;
#1081=CARTESIAN_POINT ( 'NONE',  ( -3.712013335537174572E-16, -27.06250000000000000, -6.062177826491070398 ) ) ;
#1082=EDGE_LOOP ( 'NONE', ( #8172, #4837 ) ) ;
#1086=DIRECTION ( 'NONE',  ( 0.000000000000000000, 0.000000000000000000, -1.000000000000000000 ) ) ;
#1093=AXIS2_PLACEMENT_3D ( 'NONE', #2218, #8727, #913 ) ;
#1095=CARTESIAN_POINT ( 'NONE',  ( -3.807688866302469071E-16, -29.17187499965859843, -6.218427825808274356 ) ) ;
#1096=CARTESIAN_POINT ( 'NONE',  ( 5.385316468750000141, -29.73437499965859843, -6.595110575850215044E-16 ) ) ;
#1097=STYLED_ITEM('',(#9239),#5214);
#1098=DIRECTION ( 'NONE',  ( 0.000000000000000000, 0.000000000000000000, -1.000000000000000000 ) ) ;
#1099=CARTESIAN_POINT ( 'NONE',  ( 5.385316468750001029, -29.50520833299193413, 3.109213912904135846 ) ) ;
#1101=ORIENTED_EDGE ( 'NONE', *, *, #2223, .F. ) ;
#1104=CARTESIAN_POINT ( 'NONE',  ( -2.692658234374996518, -28.81770833299193413, 4.663820869356208654 ) ) ;
#1105=VECTOR ( 'NONE', #4491, 1000.000000000000000 ) ;
#1107=CARTESIAN_POINT ( 'NONE',  ( -3.807688866302469071E-16, -28.14062499965860198, -6.218427825808274356 ) ) ;
#1116=CARTESIAN_POINT ( 'NONE',  ( 5.385316468750000141, -29.95312499965859843, -6.595110575850215044E-16 ) ) ;
#1118=CARTESIAN_POINT ( 'NONE',  ( -5.249999999999997335, -29.47916666666666785, 3.031088913245538308 ) ) ;
#1119=CARTESIAN_POINT ( 'NONE',  ( 2.692658234375002735, -28.49479166632526628, 4.663820869356205101 ) ) ;
#1120=EDGE_CURVE ( 'NONE', #2527, #2627, #6233, .T. ) ;
#1124=CARTESIAN_POINT ( 'NONE',  ( 0.000000000000000000, -50.00000000000000000, 0.000000000000000000 ) ) ;
#1128=ORIENTED_EDGE ( 'NONE', *, *, #1174, .F. ) ;
#1129=CARTESIAN_POINT ( 'NONE',  ( -5.249999999999999112, -27.97916666666666430, 3.031088913245538308 ) ) ;
#1141=CARTESIAN_POINT ( 'NONE',  ( -5.385316468750000141, -29.35937499965859843, 0.000000000000000000 ) ) ;
#1144=CARTESIAN_POINT ( 'NONE',  ( -5.385316468750000141, -29.10937499965859843, 0.000000000000000000 ) ) ;
#1146=EDGE_LOOP ( 'NONE', ( #5954, #445, #7952 ) ) ;
#1147=CARTESIAN_POINT ( 'NONE',  ( -5.250000000000000000, -27.50000000000000000, 0.000000000000000000 ) ) ;
#1149=CARTESIAN_POINT ( 'NONE',  ( 2.692658234375002735, -29.02604166632526983, 4.663820869356205101 ) ) ;
#1151=CARTESIAN_POINT ( 'NONE',  ( 1.142306659890740623E-15, -28.26562499965860553, 6.218427825808274356 ) ) ;
#1155=CARTESIAN_POINT ( 'NONE',  ( 1.406733260263395735, -27.42633545031537068, 5.250000000000000000 ) ) ;
#1160=CARTESIAN_POINT ( 'NONE',  ( -3.807688866302469071E-16, -29.14062499965860553, -6.218427825808274356 ) ) ;
#1162=DIRECTION ( 'NONE',  ( 0.000000000000000000, -1.000000000000000000, 0.000000000000000000 ) ) ;
#1163=CARTESIAN_POINT ( 'NONE',  ( 2.692658234374998738, -28.16145833299193413, -4.663820869356206877 ) ) ;
#1167=CARTESIAN_POINT ( 'NONE',  ( -4.916521616868715807E-16, -50.00000000000000000, 2.786798956483056422 ) ) ;
#1169=ADVANCED_FACE ( 'NONE', ( #6181 ), #9008, .F. ) ;
#1172=CARTESIAN_POINT ( 'NONE',  ( 5.250000000000000000, -29.10416666666666785, -3.031088913245536531 ) ) ;
#1174=EDGE_CURVE ( 'NONE', #3963, #8455, #1812, .T. ) ;
#1185=DIRECTION ( 'NONE',  ( 0.000000000000000000, -0.000000000000000000, -1.000000000000000000 ) ) ;
#1186=CARTESIAN_POINT ( 'NONE',  ( -3.807688866302469071E-16, -28.67187499965860198, -6.218427825808274356 ) ) ;
#1189=CARTESIAN_POINT ( 'NONE',  ( 1.142306659890740623E-15, -28.79687499965860198, 6.218427825808274356 ) ) ;
#1197=EDGE_CURVE ( 'NONE', #4744, #451, #2789, .T. ) ;
#1198=CARTESIAN_POINT ( 'NONE',  ( 5.385316468750000141, -29.73437499965859843, -6.595110575850215044E-16 ) ) ;
#1201=CARTESIAN_POINT ( 'NONE',  ( 5.385316468750001029, -28.47395833299193413, 3.109213912904134958 ) ) ;
#1203=CARTESIAN_POINT ( 'NONE',  ( 0.000000000000000000, -27.00000000000000000, -5.250000000000000000 ) ) ;
#1204=CARTESIAN_POINT ( 'NONE',  ( -6.972266317189433020E-16, -29.24999999931720396, -5.249999999999999112 ) ) ;
#1206=CARTESIAN_POINT ( 'NONE',  ( 5.250000000000000888, -27.39583333333333570, 3.031088913245533423 ) ) ;
#1209=LINE ( 'NONE', #4049, #340 ) ;
#1213=CARTESIAN_POINT ( 'NONE',  ( -5.250000000000000000, -29.50000000000000000, 0.000000000000000000 ) ) ;
#1214=CARTESIAN_POINT ( 'NONE',  ( 2.692658234375002735, -29.49479166632526983, 4.663820869356205101 ) ) ;
#1221=CARTESIAN_POINT ( 'NONE',  ( 5.250000000000000888, -28.89583333333333215, 3.031088913245532979 ) ) ;
#1228=EDGE_CURVE ( 'NONE', #3224, #5282, #7468, .T. ) ;
#1233=CARTESIAN_POINT ( 'NONE',  ( 1.142306659890740623E-15, -29.04687499965859843, 6.218427825808274356 ) ) ;
#1234=CARTESIAN_POINT ( 'NONE',  ( 1.142306659890740623E-15, -29.79687499965859843, 6.218427825808274356 ) ) ;
#1236=CARTESIAN_POINT ( 'NONE',  ( -5.385316468750000141, -29.35937499965859843, 0.000000000000000000 ) ) ;
#1243=CARTESIAN_POINT ( 'NONE',  ( 5.385316468750001029, -28.75520833299193413, 3.109213912904135846 ) ) ;
#1245=VECTOR ( 'NONE', #7791, 1000.000000000000000 ) ;
#1247=CARTESIAN_POINT ( 'NONE',  ( 5.385316468749999252, -27.93229166632526628, -3.109213912904138954 ) ) ;
#1258=CARTESIAN_POINT ( 'NONE',  ( -3.807688866302469071E-16, -29.39062499965860198, -6.218427825808274356 ) ) ;
#1260=CARTESIAN_POINT ( 'NONE',  ( -1.406733260263391960, -27.94866454968462932, 5.250000000000000000 ) ) ;
#1261=CARTESIAN_POINT ( 'NONE',  ( 2.692658234375002735, -27.27604166632526628, 4.663820869356205101 ) ) ;
#1263=CARTESIAN_POINT ( 'NONE',  ( 0.000000000000000000, -27.00000000000000000, 0.000000000000000000 ) ) ;
#1267=CARTESIAN_POINT ( 'NONE',  ( -5.249999999999999112, -28.22916666666666430, 3.031088913245538308 ) ) ;
#1273=DIRECTION ( 'NONE',  ( 0.000000000000000000, -1.000000000000000000, 0.000000000000000000 ) ) ;
#1276=CYLINDRICAL_SURFACE ( 'NONE', #8589, 5.250000000000000000 ) ;
#1277=CARTESIAN_POINT ( 'NONE',  ( -5.250000000000000000, -29.45833333265053611, -3.031088913245534755 ) ) ;
#1278=CARTESIAN_POINT ( 'NONE',  ( 5.385316468750000141, -29.98437499965859843, -6.595110575850215044E-16 ) ) ;
#1279=FACE_OUTER_BOUND ( 'NONE', #5439, .T. ) ;
#1283=CARTESIAN_POINT ( 'NONE',  ( 5.250000000000000000, -29.12499999999999645, -6.429395695523604153E-16 ) ) ;
#1285=CARTESIAN_POINT ( 'NONE',  ( 1.142306659890740623E-15, -29.54687499965859843, 6.218427825808274356 ) ) ;
#1287=CARTESIAN_POINT ( 'NONE',  ( 5.385316468750000141, -28.95312499965860198, -6.595110575850215044E-16 ) ) ;
#1291=( BOUNDED_CURVE ( )  B_SPLINE_CURVE ( 2, ( #2841, #2089, #2795, #8507, #7762, #34, #601, #6972, #4914 ),
 .UNSPECIFIED., .F., .F. ) 
 B_SPLINE_CURVE_WITH_KNOTS ( ( 3, 2, 2, 2, 3 ),
 ( 0.4791666666666666852, 0.4861111111111111049, 0.5000000000000000000, 0.5138888888888888395, 0.5208333333333333703 ),
 .UNSPECIFIED. ) 
 CURVE ( )  GEOMETRIC_REPRESENTATION_ITEM ( )  RATIONAL_B_SPLINE_CURVE ( ( 0.9330127018922194093, 0.9330127018922196314, 1.000000000000000000, 0.8660254037844387076, 1.000000000000000000, 0.8660254037844387076, 1.000000000000000000, 0.9330127018922187432, 0.9330127018922192983 ) ) 
 REPRESENTATION_ITEM ( '' )  );
#1295=CARTESIAN_POINT ( 'NONE',  ( 0.000000000000000000, -27.00000000000000000, 0.000000000000000000 ) ) ;
#1300=CARTESIAN_POINT ( 'NONE',  ( -5.385316468750000141, -27.35937499965860198, 0.000000000000000000 ) ) ;
#1305=ORIENTED_EDGE ( 'NONE', *, *, #4401, .F. ) ;
#1306=CARTESIAN_POINT ( 'NONE',  ( -5.250000000000000000, -28.77083333333333215, -3.031088913245534755 ) ) ;
#1318=CARTESIAN_POINT ( 'NONE',  ( -3.712013335537174572E-16, -29.49999999931720041, -6.062177826491070398 ) ) ;
#1321=CARTESIAN_POINT ( 'NONE',  ( 6.972266317189434006E-16, -27.24999999931720751, -5.250000000000000000 ) ) ;
#1326=LINE ( 'NONE', #2780, #1633 ) ;
#1328=CARTESIAN_POINT ( 'NONE',  ( 5.385316468749999252, -29.96354166632526628, -3.109213912904139399 ) ) ;
#1329=EDGE_CURVE ( 'NONE', #2527, #7225, #4224, .T. ) ;
#1331=CARTESIAN_POINT ( 'NONE',  ( 2.692658234375002735, -29.99479166632526628, 4.663820869356205101 ) ) ;
#1336=DIRECTION ( 'NONE',  ( 0.000000000000000000, 1.000000000000000000, 0.000000000000000000 ) ) ;
#1340=CARTESIAN_POINT ( 'NONE',  ( 1.406733260263393737, -27.26116454900182973, -5.250000000000000000 ) ) ;
#1347=CARTESIAN_POINT ( 'NONE',  ( 2.625000000000002220, -28.66666666666666785, 4.546633369868302132 ) ) ;
#1348=CARTESIAN_POINT ( 'NONE',  ( 5.385316468750000141, -29.70312499965859843, -6.595110575850215044E-16 ) ) ;
#1351=AXIS2_PLACEMENT_3D ( 'NONE', #2624, #3965, #1966 ) ;
#1354=CARTESIAN_POINT ( 'NONE',  ( 2.692658234375002735, -27.24479166632526628, 4.663820869356205101 ) ) ;
#1355=ORIENTED_EDGE ( 'NONE', *, *, #173, .F. ) ;
#1362=DIRECTION ( 'NONE',  ( 0.000000000000000000, -1.000000000000000000, 0.000000000000000000 ) ) ;
#1365=CARTESIAN_POINT ( 'NONE',  ( 5.250000000000000000, -29.81249999931720041, -6.429395695523604153E-16 ) ) ;
#1368=LINE ( 'NONE', #9131, #1829 ) ;
#1375=CARTESIAN_POINT ( 'NONE',  ( -5.385316468750000141, -29.07812499965860198, 0.000000000000000000 ) ) ;
#1379=CARTESIAN_POINT ( 'NONE',  ( -2.624999999999996891, -28.95833333333333215, 4.546633369868304797 ) ) ;
#1381=VECTOR ( 'NONE', #1273, 1000.000000000000000 ) ;
#1384=CARTESIAN_POINT ( 'NONE',  ( 2.624999999999998668, -27.77083333265053255, -4.546633369868303021 ) ) ;
#1389=CARTESIAN_POINT ( 'NONE',  ( 2.692658234375002735, -29.74479166632526983, 4.663820869356205101 ) ) ;
#1397=CARTESIAN_POINT ( 'NONE',  ( 5.250000000000000888, -29.64583333333333215, 3.031088913245532979 ) ) ;
#1402=CARTESIAN_POINT ( 'NONE',  ( 0.000000000000000000, -27.00000000000000000, 0.000000000000000000 ) ) ;
#1407=CARTESIAN_POINT ( 'NONE',  ( -2.624999999999996891, -29.20833333333333215, 4.546633369868304797 ) ) ;
#1408=CARTESIAN_POINT ( 'NONE',  ( 5.250000000000000000, -29.54166666598386826, -3.031088913245536531 ) ) ;
#1411=CARTESIAN_POINT ( 'NONE',  ( -5.385316468749998364, -30.08854166632526983, 3.109213912904140287 ) ) ;
#1413=ORIENTED_EDGE ( 'NONE', *, *, #4803, .T. ) ;
#1414=CARTESIAN_POINT ( 'NONE',  ( 2.161402558328724325E-14, -29.74999999931720396, -5.250000000000000000 ) ) ;
#1417=ORIENTED_EDGE ( 'NONE', *, *, #5588, .F. ) ;
#1418=CARTESIAN_POINT ( 'NONE',  ( -2.692658234374996518, -29.78645833299193413, 4.663820869356208654 ) ) ;
#1422=CARTESIAN_POINT ( 'NONE',  ( 2.161402558328724325E-14, -29.49999999931720396, -5.250000000000000000 ) ) ;
#1429=CARTESIAN_POINT ( 'NONE',  ( 2.161402558328724325E-14, -29.31250000000000000, -5.250000000000000000 ) ) ;
#1430=CARTESIAN_POINT ( 'NONE',  ( 1.142306659890740623E-15, -28.04687499965860198, 6.218427825808274356 ) ) ;
#1435=CARTESIAN_POINT ( 'NONE',  ( -2.692658234375000514, -27.36979166632526628, -4.663820869356205989 ) ) ;
#1436=ADVANCED_FACE ( 'NONE', ( #679 ), #3525, .F. ) ;
#1447=CARTESIAN_POINT ( 'NONE',  ( -5.249999999999999112, -29.66666666598386826, 3.031088913245538308 ) ) ;
#1455=CARTESIAN_POINT ( 'NONE',  ( 1.975475456537005874E-15, -29.62499999931719685, 5.250000000000000000 ) ) ;
#1458=ORIENTED_EDGE ( 'NONE', *, *, #2475, .T. ) ;
#1459=CARTESIAN_POINT ( 'NONE',  ( -3.807688866302469071E-16, -29.39062499965859843, -6.218427825808274356 ) ) ;
#1463=ORIENTED_EDGE ( 'NONE', *, *, #8661, .F. ) ;
#1467=( BOUNDED_CURVE ( )  B_SPLINE_CURVE ( 2, ( #5656, #1340, #7056, #2085, #9185, #772, #5744, #7807, #3659 ),
 .UNSPECIFIED., .F., .T. ) 
 B_SPLINE_CURVE_WITH_KNOTS ( ( 3, 2, 2, 2, 3 ),
 ( 0.02083333333333333565, 0.02777777777777777624, 0.04166666666666666435, 0.05555555555555555247, 0.06250000000000000000 ),
 .UNSPECIFIED. ) 
 CURVE ( )  GEOMETRIC_REPRESENTATION_ITEM ( )  RATIONAL_B_SPLINE_CURVE ( ( 0.9330127018922194093, 0.9330127018922194093, 1.000000000000000000, 0.8660254037844387076, 1.000000000000000000, 0.8660254037844387076, 1.000000000000000000, 0.9330127018922194093, 0.9330127018922194093 ) ) 
 REPRESENTATION_ITEM ( '' )  );
#1469=DIRECTION ( 'NONE',  ( 0.000000000000000000, 0.000000000000000000, -1.000000000000000000 ) ) ;
#1470=VECTOR ( 'NONE', #8499, 1000.000000000000000 ) ;
#1476=CARTESIAN_POINT ( 'NONE',  ( -5.385316468750001029, -28.63020833299193413, -3.109213912904136734 ) ) ;
#1481=AXIS2_PLACEMENT_3D ( 'NONE', #8184, #5149, #1012 ) ;
#1482=ORIENTED_EDGE ( 'NONE', *, *, #9169, .F. ) ;
#1483=CARTESIAN_POINT ( 'NONE',  ( 5.250000000000000000, -29.85416666666667140, -3.031088913245536531 ) ) ;
#1485=CARTESIAN_POINT ( 'NONE',  ( 2.324088772396477476E-15, -27.31250000000000000, -5.250000000000000000 ) ) ;
#1492=VECTOR ( 'NONE', #5566, 1000.000000000000114 ) ;
#1501=ORIENTED_EDGE ( 'NONE', *, *, #851, .T. ) ;
#1509=CARTESIAN_POINT ( 'NONE',  ( 1.406733260263390628, -28.17633545031536357, 5.250000000000001776 ) ) ;
#1515=CARTESIAN_POINT ( 'NONE',  ( 5.250000000000000888, -28.89583333333333215, 3.031088913245533423 ) ) ;
#1519=CARTESIAN_POINT ( 'NONE',  ( -2.692658234375000514, -27.11979166632526628, -4.663820869356205989 ) ) ;
#1522=CARTESIAN_POINT ( 'NONE',  ( 5.385316468749999252, -28.71354166632526628, -3.109213912904139399 ) ) ;
#1524=VECTOR ( 'NONE', #7266, 1000.000000000000000 ) ;
#1528=ORIENTED_EDGE ( 'NONE', *, *, #1120, .T. ) ;
#1529=CIRCLE ( 'NONE', #2124, 6.250000000000000000 ) ;
#1530=CARTESIAN_POINT ( 'NONE',  ( 5.385316468750001029, -27.22395833299193413, 3.109213912904135846 ) ) ;
#1531=( GEOMETRIC_REPRESENTATION_CONTEXT ( 3 ) GLOBAL_UNCERTAINTY_ASSIGNED_CONTEXT ( ( #996 ) ) GLOBAL_UNIT_ASSIGNED_CONTEXT ( ( #5266, #3746, #3885 ) ) REPRESENTATION_CONTEXT ( 'NONE', 'WORKASPACE' ) );
#1533=CARTESIAN_POINT ( 'NONE',  ( -5.249999999999999112, -27.27083333333333570, -3.031088913245534755 ) ) ;
#1544=CARTESIAN_POINT ( 'NONE',  ( 5.250000000000000000, -30.04166666598386826, -3.031088913245536531 ) ) ;
#1546=CARTESIAN_POINT ( 'NONE',  ( 1.975475456537005874E-15, -27.87499999931720041, 5.249999999999999112 ) ) ;
#1554=ORIENTED_EDGE ( 'NONE', *, *, #6379, .F. ) ;
#1555=ORIENTED_EDGE ( 'NONE', *, *, #1645, .F. ) ;
#1557=CARTESIAN_POINT ( 'NONE',  ( 5.250000000000000888, -28.14583333333333215, 3.031088913245533423 ) ) ;
#1559=CARTESIAN_POINT ( 'NONE',  ( -2.033577675846918216E-14, -29.37499999931720396, 5.250000000000000888 ) ) ;
#1560=EDGE_LOOP ( 'NONE', ( #8776, #8250, #6632, #1501 ) ) ;
#1563=CARTESIAN_POINT ( 'NONE',  ( 2.692658234375002735, -27.52604166632526628, 4.663820869356205101 ) ) ;
#1571=CARTESIAN_POINT ( 'NONE',  ( 2.625000000000002220, -27.35416666598386826, 4.546633369868302132 ) ) ;
#1572=CARTESIAN_POINT ( 'NONE',  ( -5.250000000000000000, -27.68749999931720396, 0.000000000000000000 ) ) ;
#1574=CARTESIAN_POINT ( 'NONE',  ( -6.420198811813273403E-16, -30.00000000000000000, 5.242490174541154069 ) ) ;
#1578=CARTESIAN_POINT ( 'NONE',  ( 2.692658234375002735, -27.99479166632526628, 4.663820869356205101 ) ) ;
#1579=DIRECTION ( 'NONE',  ( 0.000000000000000000, 0.000000000000000000, 1.000000000000000000 ) ) ;
#1580=ORIENTED_EDGE ( 'NONE', *, *, #3015, .F. ) ;
#1583=ORIENTED_EDGE ( 'NONE', *, *, #2917, .T. ) ;
#1587=CARTESIAN_POINT ( 'NONE',  ( 1.113604000661152470E-15, -27.68750000000000000, 6.062177826491070398 ) ) ;
#1592=LINE ( 'NONE', #843, #2738 ) ;
#1593=CYLINDRICAL_SURFACE ( 'NONE', #5686, 5.250000000000000000 ) ;
#1595=CARTESIAN_POINT ( 'NONE',  ( 1.406733260263395735, -28.11383544963257464, 5.250000000000000000 ) ) ;
#1598=VERTEX_POINT ( 'NONE', #7542 ) ;
#1599=CARTESIAN_POINT ( 'NONE',  ( -1.406733260263402174, -29.69866454968462222, 5.249999999999995559 ) ) ;
#1600=CARTESIAN_POINT ( 'NONE',  ( 5.385316468750001029, -27.75520833299194123, 3.109213912904134958 ) ) ;
#1603=ORIENTED_EDGE ( 'NONE', *, *, #5041, .F. ) ;
#1608=CARTESIAN_POINT ( 'NONE',  ( 5.385316468750000141, -27.48437499965860198, -6.595110575850215044E-16 ) ) ;
#1612=CARTESIAN_POINT ( 'NONE',  ( 5.385316468750001029, -27.47395833299193413, 3.109213912904134958 ) ) ;
#1617=EDGE_CURVE ( 'NONE', #6175, #7159, #6471, .T. ) ;
#1618=CARTESIAN_POINT ( 'NONE',  ( 1.113604000661152470E-15, -27.87499999931720751, 6.062177826491070398 ) ) ;
#1619=CARTESIAN_POINT ( 'NONE',  ( -1.406733260263394625, -27.73883544963256753, -5.250000000000000000 ) ) ;
#1620=AXIS2_PLACEMENT_3D ( 'NONE', #2317, #4453, #5145 ) ;
#1622=CARTESIAN_POINT ( 'NONE',  ( 5.250000000000000000, -29.06249999931720396, -6.429395695523604153E-16 ) ) ;
#1624=CARTESIAN_POINT ( 'NONE',  ( -5.385316468750001029, -28.84895833299193413, -3.109213912904136734 ) ) ;
#1626=FACE_OUTER_BOUND ( 'NONE', #4285, .T. ) ;
#1633=VECTOR ( 'NONE', #3430, 1000.000000000000114 ) ;
#1636=CARTESIAN_POINT ( 'NONE',  ( 2.624999999999998668, -27.33333333333333570, -4.546633369868303021 ) ) ;
#1639=( BOUNDED_SURFACE ( )  B_SPLINE_SURFACE ( 1, 2, ( 
 ( #3225, #7455, #889, #1081, #6750, #5302, #4427, #938, #3182, #6047, #7312, #7962, #8884, #7404, #5258, #3827, #1636, #5114, #5165, #1028, #8056, #6609, #6003, #238, #3088, #8753, #3877, #3138, #2383, #1685, #4526, #6652, #8841, #1587, #5959, #7262, #7356, #2433, #1732, #611, #6797, #2671, #5495, #6240, #3366, #1882, #6151, #1129, #4061, #8386, #5540, #2013, #6197, #9025, #8930, #3452, #474, #2578, #6281, #1267, #1924, #7501, #4838, #2715, #567, #422, #7640, #524, #4106, #6900, #3319, #4016, #8341, #8979, #6938, #1828, #8199, #2628, #4662, #1968, #4796, #7683, #4752, #3411, #9072, #1306, #5446, #3969, #7596, #4148, #5350, #1221, #6984, #2526, #3270, #8292, #6099, #5398, #8249, #4707, #7546, #1172, #6850, #3584, #4282, #8599, #2099, #5670, #737, #4374, #5713, #4239, #4965, #3496, #655, #694, #8518, #6453, #7026, #4923, #3676, #6363, #7775, #7730, #3539, #9118, #5758, #1397, #831, #6320, #2055, #7069, #87, #5624, #8556, #5005, #2763, #1483, #2805, #2184, #7862, #3, #8427, #7909, #2853 ),
 ( #2144, #5583, #2231, #8475, #7206, #5056, #4880, #1530, #1354, #2937, #4193, #7819, #4327, #9156, #1435, #7113, #6408, #7160, #46, #2895, #786, #3631, #5105, #5948, #6599, #4419, #8092, #7953, #5854, #7250, #8787, #4515, #3034, #180, #3773, #5202, #5248, #2418, #2373, #6498, #876, #229, #1769, #4604, #1578, #6642, #271, #1016, #7345, #8694, #923, #3726, #8044, #3170, #317, #5992, #970, #3817, #6549, #7443, #4463, #2324, #1068, #1721, #5899, #2279, #8831, #6687, #4557, #5153, #7393, #3124, #3864, #1672, #7301, #7997, #2467, #3078, #5291, #5809, #2984, #8739, #8647, #8141, #133, #1624, #6136, #9014, #7629, #8329, #4694, #2512, #8967, #6930, #6734, #2617, #4096, #4786, #6034, #1160, #6230, #2003, #6885, #5339, #3356, #8872, #3214, #2703, #7532, #558, #512, #1258, #6186, #2659, #4051, #4738, #1871, #9062, #5481, #1960, #4829, #3402, #410, #6838, #5532, #8188, #4004, #1817, #5434, #8376, #7674, #8280, #2567, #4649, #462, #3910, #365, #7490, #1116, #3957, #6784, #5386, #1913, #3306, #7585 ) ),
 .UNSPECIFIED., .F., .F., .F. ) 
 B_SPLINE_SURFACE_WITH_KNOTS ( ( 2, 2 ),
 ( 3, 2, 2, 2, 2, 2, 2, 2, 2, 2, 2, 2, 2, 2, 2, 2, 2, 2, 2, 2, 2, 2, 2, 2, 2, 2, 2, 2, 2, 2, 2, 2, 2, 2, 2, 2, 2, 2, 2, 2, 2, 2, 2, 2, 2, 2, 2, 2, 2, 2, 2, 2, 2, 2, 2, 2, 2, 2, 2, 2, 2, 2, 2, 2, 2, 2, 2, 2, 2, 2, 2, 2, 3 ),
 ( 0.000000000000000000, 1.000000000000000000 ),
 ( 0.000000000000000000, 0.01388888888888888812, 0.02777777777777777624, 0.04166666666666666435, 0.05555555555555555247, 0.06944444444444444753, 0.08333333333333332871, 0.09722222222222222376, 0.1111111111111111049, 0.1250000000000000000, 0.1388888888888888951, 0.1527777777777777901, 0.1666666666666666574, 0.1805555555555555525, 0.1944444444444444475, 0.2083333333333333426, 0.2222222222222222099, 0.2361111111111111049, 0.2500000000000000000, 0.2638888888888888951, 0.2777777777777777901, 0.2916666666666666852, 0.3055555555555555802, 0.3194444444444444198, 0.3333333333333333148, 0.3472222222222222099, 0.3611111111111111049, 0.3750000000000000000, 0.3888888888888888951, 0.4027777777777777901, 0.4166666666666666852, 0.4305555555555555802, 0.4444444444444444198, 0.4583333333333333148, 0.4722222222222222099, 0.4861111111111111049, 0.5000000000000000000, 0.5138888888888888395, 0.5277777777777777901, 0.5416666666666666297, 0.5555555555555555802, 0.5694444444444444198, 0.5833333333333333703, 0.5972222222222222099, 0.6111111111111111605, 0.6250000000000000000, 0.6388888888888888395, 0.6527777777777777901, 0.6666666666666666297, 0.6805555555555555802, 0.6944444444444444198, 0.7083333333333333703, 0.7222222222222222099, 0.7361111111111111605, 0.7500000000000000000, 0.7638888888888888395, 0.7777777777777777901, 0.7916666666666666297, 0.8055555555555555802, 0.8194444444444444198, 0.8333333333333333703, 0.8472222222222222099, 0.8611111111111111605, 0.8750000000000000000, 0.8888888888888888395, 0.9027777777777777901, 0.9166666666666666297, 0.9305555555555555802, 0.9444444444444444198, 0.9583333333333333703, 0.9722222222222222099, 0.9861111111111111605, 1.000000000000000000 ),
 .UNSPECIFIED. ) 
 GEOMETRIC_REPRESENTATION_ITEM ( )  RATIONAL_B_SPLINE_SURFACE ( (
 ( 1.000000000000000000, 0.8660254037844387076, 1.000000000000000000, 0.8660254037844387076, 1.000000000000000000, 0.8660254037844387076, 1.000000000000000000, 0.8660254037844387076, 1.000000000000000000, 0.8660254037844387076, 1.000000000000000000, 0.8660254037844387076, 1.000000000000000000, 0.8660254037844387076, 1.000000000000000000, 0.8660254037844387076, 1.000000000000000000, 0.8660254037844387076, 1.000000000000000000, 0.8660254037844387076, 1.000000000000000000, 0.8660254037844387076, 1.000000000000000000, 0.8660254037844387076, 1.000000000000000000, 0.8660254037844387076, 1.000000000000000000, 0.8660254037844387076, 1.000000000000000000, 0.8660254037844387076, 1.000000000000000000, 0.8660254037844387076, 1.000000000000000000, 0.8660254037844387076, 1.000000000000000000, 0.8660254037844387076, 1.000000000000000000, 0.8660254037844387076, 1.000000000000000000, 0.8660254037844387076, 1.000000000000000000, 0.8660254037844387076, 1.000000000000000000, 0.8660254037844387076, 1.000000000000000000, 0.8660254037844387076, 1.000000000000000000, 0.8660254037844387076, 1.000000000000000000, 0.8660254037844387076, 1.000000000000000000, 0.8660254037844387076, 1.000000000000000000, 0.8660254037844387076, 1.000000000000000000, 0.8660254037844387076, 1.000000000000000000, 0.8660254037844387076, 1.000000000000000000, 0.8660254037844387076, 1.000000000000000000, 0.8660254037844387076, 1.000000000000000000, 0.8660254037844387076, 1.000000000000000000, 0.8660254037844387076, 1.000000000000000000, 0.8660254037844387076, 1.000000000000000000, 0.8660254037844387076, 1.000000000000000000, 0.8660254037844387076, 1.000000000000000000, 0.8660254037844387076, 1.000000000000000000, 0.8660254037844387076, 1.000000000000000000, 0.8660254037844387076, 1.000000000000000000, 0.8660254037844387076, 1.000000000000000000, 0.8660254037844387076, 1.000000000000000000, 0.8660254037844387076, 1.000000000000000000, 0.8660254037844387076, 1.000000000000000000, 0.8660254037844387076, 1.000000000000000000, 0.8660254037844387076, 1.000000000000000000, 0.8660254037844387076, 1.000000000000000000, 0.8660254037844387076, 1.000000000000000000, 0.8660254037844387076, 1.000000000000000000, 0.8660254037844387076, 1.000000000000000000, 0.8660254037844387076, 1.000000000000000000, 0.8660254037844387076, 1.000000000000000000, 0.8660254037844387076, 1.000000000000000000, 0.8660254037844387076, 1.000000000000000000, 0.8660254037844387076, 1.000000000000000000, 0.8660254037844387076, 1.000000000000000000, 0.8660254037844387076, 1.000000000000000000, 0.8660254037844387076, 1.000000000000000000, 0.8660254037844387076, 1.000000000000000000, 0.8660254037844387076, 1.000000000000000000, 0.8660254037844387076, 1.000000000000000000, 0.8660254037844387076, 1.000000000000000000, 0.8660254037844387076, 1.000000000000000000, 0.8660254037844387076, 1.000000000000000000, 0.8660254037844387076, 1.000000000000000000, 0.8660254037844387076, 1.000000000000000000, 0.8660254037844387076, 1.000000000000000000, 0.8660254037844387076, 1.000000000000000000, 0.8660254037844387076, 1.000000000000000000, 0.8660254037844387076, 1.000000000000000000, 0.8660254037844387076, 1.000000000000000000, 0.8660254037844387076, 1.000000000000000000, 0.8660254037844387076, 1.000000000000000000),
 ( 1.000000000000000000, 0.8660254037844387076, 1.000000000000000000, 0.8660254037844387076, 1.000000000000000000, 0.8660254037844387076, 1.000000000000000000, 0.8660254037844387076, 1.000000000000000000, 0.8660254037844387076, 1.000000000000000000, 0.8660254037844387076, 1.000000000000000000, 0.8660254037844387076, 1.000000000000000000, 0.8660254037844387076, 1.000000000000000000, 0.8660254037844387076, 1.000000000000000000, 0.8660254037844387076, 1.000000000000000000, 0.8660254037844387076, 1.000000000000000000, 0.8660254037844387076, 1.000000000000000000, 0.8660254037844387076, 1.000000000000000000, 0.8660254037844387076, 1.000000000000000000, 0.8660254037844387076, 1.000000000000000000, 0.8660254037844387076, 1.000000000000000000, 0.8660254037844387076, 1.000000000000000000, 0.8660254037844387076, 1.000000000000000000, 0.8660254037844387076, 1.000000000000000000, 0.8660254037844387076, 1.000000000000000000, 0.8660254037844387076, 1.000000000000000000, 0.8660254037844387076, 1.000000000000000000, 0.8660254037844387076, 1.000000000000000000, 0.8660254037844387076, 1.000000000000000000, 0.8660254037844387076, 1.000000000000000000, 0.8660254037844387076, 1.000000000000000000, 0.8660254037844387076, 1.000000000000000000, 0.8660254037844387076, 1.000000000000000000, 0.8660254037844387076, 1.000000000000000000, 0.8660254037844387076, 1.000000000000000000, 0.8660254037844387076, 1.000000000000000000, 0.8660254037844387076, 1.000000000000000000, 0.8660254037844387076, 1.000000000000000000, 0.8660254037844387076, 1.000000000000000000, 0.8660254037844387076, 1.000000000000000000, 0.8660254037844387076, 1.000000000000000000, 0.8660254037844387076, 1.000000000000000000, 0.8660254037844387076, 1.000000000000000000, 0.8660254037844387076, 1.000000000000000000, 0.8660254037844387076, 1.000000000000000000, 0.8660254037844387076, 1.000000000000000000, 0.8660254037844387076, 1.000000000000000000, 0.8660254037844387076, 1.000000000000000000, 0.8660254037844387076, 1.000000000000000000, 0.8660254037844387076, 1.000000000000000000, 0.8660254037844387076, 1.000000000000000000, 0.8660254037844387076, 1.000000000000000000, 0.8660254037844387076, 1.000000000000000000, 0.8660254037844387076, 1.000000000000000000, 0.8660254037844387076, 1.000000000000000000, 0.8660254037844387076, 1.000000000000000000, 0.8660254037844387076, 1.000000000000000000, 0.8660254037844387076, 1.000000000000000000, 0.8660254037844387076, 1.000000000000000000, 0.8660254037844387076, 1.000000000000000000, 0.8660254037844387076, 1.000000000000000000, 0.8660254037844387076, 1.000000000000000000, 0.8660254037844387076, 1.000000000000000000, 0.8660254037844387076, 1.000000000000000000, 0.8660254037844387076, 1.000000000000000000, 0.8660254037844387076, 1.000000000000000000, 0.8660254037844387076, 1.000000000000000000, 0.8660254037844387076, 1.000000000000000000, 0.8660254037844387076, 1.000000000000000000, 0.8660254037844387076, 1.000000000000000000, 0.8660254037844387076, 1.000000000000000000, 0.8660254037844387076, 1.000000000000000000, 0.8660254037844387076, 1.000000000000000000, 0.8660254037844387076, 1.000000000000000000, 0.8660254037844387076, 1.000000000000000000, 0.8660254037844387076, 1.000000000000000000, 0.8660254037844387076, 1.000000000000000000) ) ) 
 REPRESENTATION_ITEM ( '' )  SURFACE ( )  );
#1645=EDGE_CURVE ( 'NONE', #2851, #105, #3332, .T. ) ;
#1652=CARTESIAN_POINT ( 'NONE',  ( -5.385316468750000141, -27.09374999965859843, 0.000000000000000000 ) ) ;
#1653=CARTESIAN_POINT ( 'NONE',  ( 5.385316468749999252, -27.96354166632526628, -3.109213912904138954 ) ) ;
#1659=EDGE_CURVE ( 'NONE', #3226, #1074, #5924, .T. ) ;
#1660=CARTESIAN_POINT ( 'NONE',  ( -2.692658234375000514, -27.65104166632526628, -4.663820869356205989 ) ) ;
#1663=CARTESIAN_POINT ( 'NONE',  ( 5.385316468750000141, -27.45312499965860198, -6.595110575850215044E-16 ) ) ;
#1665=CARTESIAN_POINT ( 'NONE',  ( -1.406733260263393070, -27.48883544963257108, -5.250000000000000888 ) ) ;
#1667=CARTESIAN_POINT ( 'NONE',  ( -3.712013335537174572E-16, -27.74999999931720396, -6.062177826491070398 ) ) ;
#1668=CARTESIAN_POINT ( 'NONE',  ( -1.406733260263394625, -27.05133545031536713, -5.250000000000000000 ) ) ;
#1670=CARTESIAN_POINT ( 'NONE',  ( 1.406733260263385521, -29.86383544963257108, 5.250000000000006217 ) ) ;
#1672=CARTESIAN_POINT ( 'NONE',  ( -5.385316468750001029, -28.59895833299193413, -3.109213912904136734 ) ) ;
#1674=DIRECTION ( 'NONE',  ( 0.000000000000000000, -1.000000000000000000, 0.000000000000000000 ) ) ;
#1676=CARTESIAN_POINT ( 'NONE',  ( -2.692658234374996518, -27.78645833299193413, 4.663820869356208654 ) ) ;
#1679=ORIENTED_EDGE ( 'NONE', *, *, #313, .T. ) ;
#1685=CARTESIAN_POINT ( 'NONE',  ( 5.250000000000000000, -27.60416666666666785, -3.031088913245536531 ) ) ;
#1687=CARTESIAN_POINT ( 'NONE',  ( 2.624999999999998668, -30.02083333265053611, -4.546633369868303021 ) ) ;
#1700=CARTESIAN_POINT ( 'NONE',  ( -3.807688866302469071E-16, -27.42187499965860198, -6.218427825808274356 ) ) ;
#1703=CARTESIAN_POINT ( 'NONE',  ( 5.385316468749999252, -27.96354166632526628, -3.109213912904139399 ) ) ;
#1707=CARTESIAN_POINT ( 'NONE',  ( -2.692658234374996518, -28.31770833299193413, 4.663820869356208654 ) ) ;
#1712=CARTESIAN_POINT ( 'NONE',  ( -5.250000000000000000, -27.43749999931720396, 0.000000000000000000 ) ) ;
#1713=CARTESIAN_POINT ( 'NONE',  ( 5.250000000000000000, -27.81249999931720396, -6.429395695523604153E-16 ) ) ;
#1717=FACE_OUTER_BOUND ( 'NONE', #1005, .T. ) ;
#1718=DIRECTION ( 'NONE',  ( 0.000000000000000000, -1.000000000000000000, 0.000000000000000000 ) ) ;
#1721=CARTESIAN_POINT ( 'NONE',  ( -3.807688866302469071E-16, -28.39062499965859843, -6.218427825808274356 ) ) ;
#1725=CARTESIAN_POINT ( 'NONE',  ( 2.692658234375002735, -27.74479166632526628, 4.663820869356205101 ) ) ;
#1727=ORIENTED_EDGE ( 'NONE', *, *, #6142, .F. ) ;
#1732=CARTESIAN_POINT ( 'NONE',  ( -2.625000000000000444, -27.79166666666666430, -4.546633369868303021 ) ) ;
#1733=ORIENTED_EDGE ( 'NONE', *, *, #2223, .T. ) ;
#1737=CARTESIAN_POINT ( 'NONE',  ( 2.161402558328724325E-14, -29.49999999931720396, -5.250000000000000000 ) ) ;
#1747=CARTESIAN_POINT ( 'NONE',  ( -5.385316468750000141, -28.85937499965860198, 0.000000000000000000 ) ) ;
#1751=CARTESIAN_POINT ( 'NONE',  ( -5.385316468749998364, -27.83854166632526628, 3.109213912904140287 ) ) ;
#1756=CARTESIAN_POINT ( 'NONE',  ( -3.807688866302469071E-16, -27.67187499965859843, -6.218427825808274356 ) ) ;
#1757=ORIENTED_EDGE ( 'NONE', *, *, #2513, .F. ) ;
#1758=CARTESIAN_POINT ( 'NONE',  ( 1.142306659890740623E-15, -28.76562499965860553, 6.218427825808274356 ) ) ;
#1763=CARTESIAN_POINT ( 'NONE',  ( -3.712013335537174572E-16, -27.99999999931720396, -6.062177826491070398 ) ) ;
#1764=CARTESIAN_POINT ( 'NONE',  ( -5.250000000000000000, -27.00000000000000000, 0.000000000000000000 ) ) ;
#1769=CARTESIAN_POINT ( 'NONE',  ( 5.385316468750000141, -27.95312499965860198, -6.595110575850215044E-16 ) ) ;
#1773=CARTESIAN_POINT ( 'NONE',  ( 5.385316468750001029, -28.22395833299193058, 3.109213912904135846 ) ) ;
#1786=VECTOR ( 'NONE', #5974, 1000.000000000000000 ) ;
#1795=CARTESIAN_POINT ( 'NONE',  ( 5.249999999999999112, -27.85416666666666430, -3.031088913245536975 ) ) ;
#1796=CARTESIAN_POINT ( 'NONE',  ( -5.385316468750000141, -28.60937499965860198, 0.000000000000000000 ) ) ;
#1798=CARTESIAN_POINT ( 'NONE',  ( -5.385316468749998364, -29.58854166632527694, 3.109213912904140287 ) ) ;
#1800=AXIS2_PLACEMENT_3D ( 'NONE', #2096, #4960, #5001 ) ;
#1803=CARTESIAN_POINT ( 'NONE',  ( -5.385316468750001029, -29.63020833299193768, -3.109213912904136734 ) ) ;
#1808=CARTESIAN_POINT ( 'NONE',  ( -5.385316468750001029, -27.84895833299193413, -3.109213912904136734 ) ) ;
#1812=LINE ( 'NONE', #6268, #6422 ) ;
#1817=CARTESIAN_POINT ( 'NONE',  ( 5.385316468750001029, -29.72395833299193413, 3.109213912904135846 ) ) ;
#1819=DIRECTION ( 'NONE',  ( 0.000000000000000000, 0.000000000000000000, -1.000000000000000000 ) ) ;
#1820=CARTESIAN_POINT ( 'NONE',  ( 2.692658234374998738, -28.66145833299193413, -4.663820869356206877 ) ) ;
#1828=CARTESIAN_POINT ( 'NONE',  ( -3.712013335537174572E-16, -28.56249999999999645, -6.062177826491070398 ) ) ;
#1829=VECTOR ( 'NONE', #8570, 1000.000000000000114 ) ;
#1837=CARTESIAN_POINT ( 'NONE',  ( -2.625000000000000444, -29.22916666598386826, -4.546633369868303021 ) ) ;
#1839=AXIS2_PLACEMENT_3D ( 'NONE', #1295, #9147, #511 ) ;
#1840=AXIS2_PLACEMENT_3D ( 'NONE', #8431, #4287, #5630 ) ;
#1846=LINE ( 'NONE', #8117, #3782 ) ;
#1847=CARTESIAN_POINT ( 'NONE',  ( 2.692658234375002735, -28.77604166632526628, 4.663820869356205101 ) ) ;
#1848=CARTESIAN_POINT ( 'NONE',  ( 0.000000000000000000, -27.00000000000000000, -5.250000000000000000 ) ) ;
#1850=CARTESIAN_POINT ( 'NONE',  ( 2.324088772396477476E-15, -27.49999999931720751, -5.250000000000000000 ) ) ;
#1851=CARTESIAN_POINT ( 'NONE',  ( 5.385316468750001029, -30.00520833299193768, 3.109213912904135846 ) ) ;
#1856=CARTESIAN_POINT ( 'NONE',  ( 2.692658234374998738, -28.69270833299193413, -4.663820869356206877 ) ) ;
#1860=CARTESIAN_POINT ( 'NONE',  ( -2.692658234374996518, -27.78645833299193413, 4.663820869356208654 ) ) ;
#1863=EDGE_CURVE ( 'NONE', #610, #27, #607, .T. ) ;
#1867=ADVANCED_FACE ( 'NONE', ( #8196 ), #5538, .F. ) ;
#1869=ORIENTED_EDGE ( 'NONE', *, *, #7652, .T. ) ;
#1871=CARTESIAN_POINT ( 'NONE',  ( 2.692658234375002735, -29.49479166632526983, 4.663820869356205101 ) ) ;
#1874=CARTESIAN_POINT ( 'NONE',  ( -3.807688866302469071E-16, -28.89062499965860198, -6.218427825808274356 ) ) ;
#1877=CARTESIAN_POINT ( 'NONE',  ( -2.624999999999996891, -30.14583333265053611, 4.546633369868304797 ) ) ;
#1881=SURFACE_STYLE_FILL_AREA ( #5445 ) ;
#1882=CARTESIAN_POINT ( 'NONE',  ( 1.113604000661152470E-15, -27.93750000000000000, 6.062177826491070398 ) ) ;
#1893=CARTESIAN_POINT ( 'NONE',  ( -5.385316468750001029, -29.13020833299193058, -3.109213912904136734 ) ) ;
#1895=CARTESIAN_POINT ( 'NONE',  ( 1.142306659890740623E-15, -29.29687499965860198, 6.218427825808274356 ) ) ;
#1900=CARTESIAN_POINT ( 'NONE',  ( -5.385316468750000141, -28.85937499965860198, 0.000000000000000000 ) ) ;
#1902=CARTESIAN_POINT ( 'NONE',  ( 5.385316468750001029, -28.22395833299193413, 3.109213912904134958 ) ) ;
#1904=DIRECTION ( 'NONE',  ( 0.000000000000000000, -1.000000000000000000, 0.000000000000000000 ) ) ;
#1908=CARTESIAN_POINT ( 'NONE',  ( -6.972266317189433020E-16, -28.49999999931720041, -5.250000000000000000 ) ) ;
#1913=CARTESIAN_POINT ( 'NONE',  ( -2.692658234374996518, -30.03645833299193413, 4.663820869356208654 ) ) ;
#1916=CARTESIAN_POINT ( 'NONE',  ( -2.624999999999996891, -29.45833333333333215, 4.546633369868304797 ) ) ;
#1917=CARTESIAN_POINT ( 'NONE',  ( -2.692658234374996518, -30.03645833299193413, 4.663820869356208654 ) ) ;
#1920=CARTESIAN_POINT ( 'NONE',  ( 1.406733300191166602, -30.01116454931871402, -5.249999976947688829 ) ) ;
#1923=EDGE_LOOP ( 'NONE', ( #2916, #7141, #653, #4705 ) ) ;
#1924=CARTESIAN_POINT ( 'NONE',  ( -5.250000000000000000, -28.25000000000000000, 0.000000000000000000 ) ) ;
#1925=ORIENTED_EDGE ( 'NONE', *, *, #6506, .T. ) ;
#1937=CARTESIAN_POINT ( 'NONE',  ( -5.385316468750000141, -28.35937499965860198, 0.000000000000000000 ) ) ;
#1939=CARTESIAN_POINT ( 'NONE',  ( 5.385316468750000141, -29.98437499965859843, -6.595110575850215044E-16 ) ) ;
#1946=CARTESIAN_POINT ( 'NONE',  ( 5.385316468750000141, -28.98437499965859843, -6.595110575850215044E-16 ) ) ;
#1948=CARTESIAN_POINT ( 'NONE',  ( 2.692658234374998738, -28.66145833299193413, -4.663820869356206877 ) ) ;
#1952=( BOUNDED_CURVE ( )  B_SPLINE_CURVE ( 2, ( #7631, #3960, #9065, #5484, #3358, #7677, #4006, #4740, #9016 ),
 .UNSPECIFIED., .F., .F. ) 
 B_SPLINE_CURVE_WITH_KNOTS ( ( 3, 2, 2, 2, 3 ),
 ( 0.4375000000000000000, 0.4444444444444444198, 0.4583333333333333148, 0.4722222222222222099, 0.4791666666666666852 ),
 .UNSPECIFIED. ) 
 CURVE ( )  GEOMETRIC_REPRESENTATION_ITEM ( )  RATIONAL_B_SPLINE_CURVE ( ( 0.9330127018922194093, 0.9330127018922194093, 1.000000000000000000, 0.8660254037844387076, 1.000000000000000000, 0.8660254037844387076, 1.000000000000000000, 0.9330127018922190762, 0.9330127018922194093 ) ) 
 REPRESENTATION_ITEM ( '' )  );
#1955=CARTESIAN_POINT ( 'NONE',  ( 1.406733260263403507, -28.82366454968462222, -5.249999999999994671 ) ) ;
#1956=AXIS2_PLACEMENT_3D ( 'NONE', #1124, #8287, #2575 ) ;
#1958=DIRECTION ( 'NONE',  ( 0.000000000000000000, 0.000000000000000000, -1.000000000000000000 ) ) ;
#1960=CARTESIAN_POINT ( 'NONE',  ( -5.385316468749998364, -29.55729166632526983, 3.109213912904140287 ) ) ;
#1963=CARTESIAN_POINT ( 'NONE',  ( -5.385316468750001029, -27.13020833299193413, -3.109213912904136734 ) ) ;
#1965=CARTESIAN_POINT ( 'NONE',  ( -5.250000000000000000, -30.18749999931720041, 0.000000000000000000 ) ) ;
#1966=DIRECTION ( 'NONE',  ( 0.000000000000000000, 0.000000000000000000, -1.000000000000000000 ) ) ;
#1968=CARTESIAN_POINT ( 'NONE',  ( 5.250000000000000888, -28.64583333333332860, 3.031088913245532979 ) ) ;
#1973=LINE ( 'NONE', #8985, #1381 ) ;
#1978=CARTESIAN_POINT ( 'NONE',  ( -3.712013335537174572E-16, -28.99999999931720751, -6.062177826491070398 ) ) ;
#1979=LINE ( 'NONE', #1848, #3459 ) ;
#1981=CARTESIAN_POINT ( 'NONE',  ( -5.385316468750001029, -29.88020833299193413, -3.109213912904136734 ) ) ;
#1984=AXIS2_PLACEMENT_3D ( 'NONE', #2199, #5726, #3555 ) ;
#1989=CARTESIAN_POINT ( 'NONE',  ( -2.692658234375000514, -28.90104166632526983, -4.663820869356205989 ) ) ;
#1992=ORIENTED_EDGE ( 'NONE', *, *, #2626, .F. ) ;
#1995=DIRECTION ( 'NONE',  ( 0.000000000000000000, 0.000000000000000000, -1.000000000000000000 ) ) ;
#1996=CIRCLE ( 'NONE', #506, 5.250000000000000000 ) ;
#2003=CARTESIAN_POINT ( 'NONE',  ( 5.385316468749999252, -29.18229166632526983, -3.109213912904139399 ) ) ;
#2006=CARTESIAN_POINT ( 'NONE',  ( 1.045839947578414884E-14, -28.06249999999999289, -5.250000000000000000 ) ) ;
#2007=CARTESIAN_POINT ( 'NONE',  ( 5.385316468750000141, -27.23437499965860198, -6.595110575850215044E-16 ) ) ;
#2013=CARTESIAN_POINT ( 'NONE',  ( -3.712013335537174572E-16, -28.06250000000000000, -6.062177826491070398 ) ) ;
#2022=CARTESIAN_POINT ( 'NONE',  ( 0.000000000000000000, -27.00000000000000000, 0.000000000000000000 ) ) ;
#2023=CARTESIAN_POINT ( 'NONE',  ( -5.250000000000000000, -28.68749999931720396, 0.000000000000000000 ) ) ;
#2033=CARTESIAN_POINT ( 'NONE',  ( 2.692658234374998738, -29.94270833299193413, -4.663820869356206877 ) ) ;
#2034=ORIENTED_EDGE ( 'NONE', *, *, #3389, .F. ) ;
#2035=CARTESIAN_POINT ( 'NONE',  ( -5.385316468749998364, -29.55729166632526983, 3.109213912904140287 ) ) ;
#2037=CARTESIAN_POINT ( 'NONE',  ( 6.429395695523604153E-16, -27.00000000000000000, 5.250000000000000000 ) ) ;
#2038=CARTESIAN_POINT ( 'NONE',  ( -5.249999999999997335, -28.97916666666666430, 3.031088913245538308 ) ) ;
#2040=DIRECTION ( 'NONE',  ( 0.000000000000000000, 0.000000000000000000, -1.000000000000000000 ) ) ;
#2042=CARTESIAN_POINT ( 'NONE',  ( 1.406733260263390628, -28.36383544963256753, 5.250000000000001776 ) ) ;
#2047=CARTESIAN_POINT ( 'NONE',  ( 2.692658234374998738, -29.16145833299193413, -4.663820869356206877 ) ) ;
#2053=( GEOMETRIC_REPRESENTATION_CONTEXT ( 3 ) GLOBAL_UNCERTAINTY_ASSIGNED_CONTEXT ( ( #860 ) ) GLOBAL_UNIT_ASSIGNED_CONTEXT ( ( #473, #3318, #6899 ) ) REPRESENTATION_CONTEXT ( 'NONE', 'WORKASPACE' ) );
#2055=CARTESIAN_POINT ( 'NONE',  ( -2.624999999999996891, -29.70833333333333215, 4.546633369868304797 ) ) ;
#2063=CARTESIAN_POINT ( 'NONE',  ( -5.250000000000000000, -29.18749999931720396, 0.000000000000000000 ) ) ;
#2068=EDGE_LOOP ( 'NONE', ( #4434, #51, #3698, #1603 ) ) ;
#2070=CARTESIAN_POINT ( 'NONE',  ( -5.249999999999999112, -29.70833333265053611, -3.031088913245534755 ) ) ;
#2076=CARTESIAN_POINT ( 'NONE',  ( -2.692658234375000514, -29.11979166632526983, -4.663820869356205989 ) ) ;
#2078=LINE ( 'NONE', #9180, #1470 ) ;
#2085=CARTESIAN_POINT ( 'NONE',  ( 5.249999999999999112, -27.29166666598386826, -3.031088913245536975 ) ) ;
#2089=CARTESIAN_POINT ( 'NONE',  ( -1.406733260263397289, -28.63616454900182973, 5.249999999999997335 ) ) ;
#2092=CARTESIAN_POINT ( 'NONE',  ( 5.250000000000000888, -28.64583333333332860, 3.031088913245533423 ) ) ;
#2093=CARTESIAN_POINT ( 'NONE',  ( -5.385316468750000141, -29.07812499965860198, 0.000000000000000000 ) ) ;
#2096=CARTESIAN_POINT ( 'NONE',  ( 0.000000000000000000, -50.00000000000000000, 0.000000000000000000 ) ) ;
#2098=ORIENTED_EDGE ( 'NONE', *, *, #6789, .T. ) ;
#2099=CARTESIAN_POINT ( 'NONE',  ( -2.624999999999996891, -29.20833333333333215, 4.546633369868304797 ) ) ;
#2104=CARTESIAN_POINT ( 'NONE',  ( -5.385316468750000141, -30.09374999965860198, 0.000000000000000000 ) ) ;
#2107=CARTESIAN_POINT ( 'NONE',  ( -5.250000000000000000, -29.20833333265053611, -3.031088913245534755 ) ) ;
#2109=CARTESIAN_POINT ( 'NONE',  ( 0.000000000000000000, -27.00000000000000000, -5.250000000000000000 ) ) ;
#2115=CARTESIAN_POINT ( 'NONE',  ( 1.975475456537005874E-15, -28.87499999931720396, 5.250000000000000000 ) ) ;
#2119=CARTESIAN_POINT ( 'NONE',  ( 5.385316468750001029, -28.97395833299193413, 3.109213912904134958 ) ) ;
#2123=CARTESIAN_POINT ( 'NONE',  ( -1.406733260263394625, -29.05133545031537068, -5.250000000000000000 ) ) ;
#2124=AXIS2_PLACEMENT_3D ( 'NONE', #5746, #4267, #3573 ) ;
#2127=CARTESIAN_POINT ( 'NONE',  ( -3.807688866302469071E-16, -27.17187499965860198, -6.218427825808274356 ) ) ;
#2128=EDGE_CURVE ( 'NONE', #7091, #4744, #5796, .T. ) ;
#2130=CARTESIAN_POINT ( 'NONE',  ( -5.250000000000000000, -28.18749999931720396, 0.000000000000000000 ) ) ;
#2136=CARTESIAN_POINT ( 'NONE',  ( 5.385316468750001029, -28.50520833299193058, 3.109213912904135846 ) ) ;
#2144=CARTESIAN_POINT ( 'NONE',  ( -5.385316468750000141, -27.07812499965860198, 0.000000000000000000 ) ) ;
#2150=CARTESIAN_POINT ( 'NONE',  ( 2.625000000000002220, -29.41666666666666785, 4.546633369868302132 ) ) ;
#2155=CARTESIAN_POINT ( 'NONE',  ( 2.624999999999998668, -29.77083333265053611, -4.546633369868303021 ) ) ;
#2161=CARTESIAN_POINT ( 'NONE',  ( 1.406733260263385521, -29.17633545031537423, 5.250000000000006217 ) ) ;
#2163=ORIENTED_EDGE ( 'NONE', *, *, #7789, .T. ) ;
#2165=CYLINDRICAL_SURFACE ( 'NONE', #7932, 5.250000000000000000 ) ;
#2169=CARTESIAN_POINT ( 'NONE',  ( -9.180150650966086169E-15, -28.37499999931720041, 5.249999999999999112 ) ) ;
#2171=CARTESIAN_POINT ( 'NONE',  ( 2.624999999999998668, -28.83333333333333215, -4.546633369868303021 ) ) ;
#2178=CARTESIAN_POINT ( 'NONE',  ( 5.385316468749999252, -28.21354166632526983, -3.109213912904139399 ) ) ;
#2184=CARTESIAN_POINT ( 'NONE',  ( 5.250000000000000888, -29.89583333333333215, 3.031088913245532979 ) ) ;
#2199=CARTESIAN_POINT ( 'NONE',  ( 0.000000000000000000, -30.00000000000000000, 0.000000000000000000 ) ) ;
#2202=VERTEX_POINT ( 'NONE', #4732 ) ;
#2207=ORIENTED_EDGE ( 'NONE', *, *, #6586, .F. ) ;
#2209=CARTESIAN_POINT ( 'NONE',  ( 2.692658234375002735, -27.27604166632526628, 4.663820869356205101 ) ) ;
#2212=VERTEX_POINT ( 'NONE', #1204 ) ;
#2215=FACE_OUTER_BOUND ( 'NONE', #6032, .T. ) ;
#2218=CARTESIAN_POINT ( 'NONE',  ( 0.000000000000000000, -27.00000000000000000, 0.000000000000000000 ) ) ;
#2222=CARTESIAN_POINT ( 'NONE',  ( -2.692658234375000514, -28.65104166632526628, -4.663820869356205989 ) ) ;
#2223=EDGE_CURVE ( 'NONE', #8584, #6343, #2555, .T. ) ;
#2231=CARTESIAN_POINT ( 'NONE',  ( -2.692658234375000514, -27.11979166632526628, -4.663820869356205989 ) ) ;
#2233=CARTESIAN_POINT ( 'NONE',  ( -3.807688866302469071E-16, -27.14062499965860198, -6.218427825808274356 ) ) ;
#2236=ORIENTED_EDGE ( 'NONE', *, *, #5626, .F. ) ;
#2238=DIRECTION ( 'NONE',  ( -0.000000000000000000, 1.000000000000000000, -0.000000000000000000 ) ) ;
#2245=CARTESIAN_POINT ( 'NONE',  ( -2.625000000000000444, -29.97916666598387181, -4.546633369868303021 ) ) ;
#2246=CARTESIAN_POINT ( 'NONE',  ( -5.249999999999997335, -28.22916666666666430, 3.031088913245538308 ) ) ;
#2250=DIRECTION ( 'NONE',  ( 0.000000000000000000, -1.000000000000000000, 0.000000000000000000 ) ) ;
#2253=EDGE_CURVE ( 'NONE', #8014, #3220, #5474, .T. ) ;
#2254=ORIENTED_EDGE ( 'NONE', *, *, #7167, .F. ) ;
#2255=ORIENTED_EDGE ( 'NONE', *, *, #4966, .F. ) ;
#2257=CARTESIAN_POINT ( 'NONE',  ( -2.692658234375000514, -27.90104166632526628, -4.663820869356205989 ) ) ;
#2263=CARTESIAN_POINT ( 'NONE',  ( 5.385316468750001029, -28.50520833299193058, 3.109213912904135846 ) ) ;
#2267=CARTESIAN_POINT ( 'NONE',  ( 5.249999999999999112, -28.79166666598386826, -3.031088913245536975 ) ) ;
#2269=CARTESIAN_POINT ( 'NONE',  ( -2.033577675846918216E-14, -29.37499999931720396, 5.250000000000000888 ) ) ;
#2271=AXIS2_PLACEMENT_3D ( 'NONE', #198, #4065, #1086 ) ;
#2272=CARTESIAN_POINT ( 'NONE',  ( 5.250000000000000000, -28.31249999931720396, -6.429395695523604153E-16 ) ) ;
#2275=CARTESIAN_POINT ( 'NONE',  ( 5.250000000000000888, -29.83333333265053611, 3.031088913245533423 ) ) ;
#2279=CARTESIAN_POINT ( 'NONE',  ( 5.385316468749999252, -28.43229166632526983, -3.109213912904139399 ) ) ;
#2280=CARTESIAN_POINT ( 'NONE',  ( 2.161402558328724325E-14, -28.81250000000000355, -5.250000000000000000 ) ) ;
#2282=CARTESIAN_POINT ( 'NONE',  ( -2.625000000000000444, -27.29166666666666430, -4.546633369868303021 ) ) ;
#2284=ORIENTED_EDGE ( 'NONE', *, *, #6586, .T. ) ;
#2291=( BOUNDED_CURVE ( )  B_SPLINE_CURVE ( 2, ( #4540, #7372, #8768, #5131, #7327, #812, #252, #7938, #1559 ),
 .UNSPECIFIED., .F., .F. ) 
 B_SPLINE_CURVE_WITH_KNOTS ( ( 3, 2, 2, 2, 3 ),
 ( 0.6875000000000000000, 0.6944444444444444198, 0.7083333333333333703, 0.7222222222222222099, 0.7291666666666667407 ),
 .UNSPECIFIED. ) 
 CURVE ( )  GEOMETRIC_REPRESENTATION_ITEM ( )  RATIONAL_B_SPLINE_CURVE ( ( 0.9330127018922194093, 0.9330127018922194093, 1.000000000000000000, 0.8660254037844387076, 1.000000000000000000, 0.8660254037844387076, 1.000000000000000000, 0.9330127018922187432, 0.9330127018922192983 ) ) 
 REPRESENTATION_ITEM ( '' )  );
#2293=PLANE ( 'NONE',  #4015 ) ;
#2294=CARTESIAN_POINT ( 'NONE',  ( -6.972266317189433020E-16, -28.31249999999999645, -5.250000000000000000 ) ) ;
#2306=CARTESIAN_POINT ( 'NONE',  ( 5.385316468750000141, -27.73437499965860198, -6.595110575850215044E-16 ) ) ;
#2312=CARTESIAN_POINT ( 'NONE',  ( -2.692658234375000514, -28.40104166632526628, -4.663820869356205989 ) ) ;
#2315=CARTESIAN_POINT ( 'NONE',  ( -5.385316468749998364, -27.30729166632526272, 3.109213912904140287 ) ) ;
#2317=CARTESIAN_POINT ( 'NONE',  ( 0.000000000000000000, -27.00000000000000000, 0.000000000000000000 ) ) ;
#2319=CARTESIAN_POINT ( 'NONE',  ( 1.113604000661152470E-15, -28.12499999931720041, 6.062177826491070398 ) ) ;
#2320=CARTESIAN_POINT ( 'NONE',  ( 2.625000000000002220, -27.66666666666666430, 4.546633369868302132 ) ) ;
#2324=CARTESIAN_POINT ( 'NONE',  ( -5.385316468750001029, -28.34895833299193058, -3.109213912904136734 ) ) ;
#2327=DIRECTION ( 'NONE',  ( 0.000000000000000000, -1.000000000000000000, 0.000000000000000000 ) ) ;
#2328=ORIENTED_EDGE ( 'NONE', *, *, #6043, .F. ) ;
#2331=VERTEX_POINT ( 'NONE', #8412 ) ;
#2335=CARTESIAN_POINT ( 'NONE',  ( 2.625000000000002220, -30.10416666598386826, 4.546633369868302132 ) ) ;
#2337=CARTESIAN_POINT ( 'NONE',  ( -5.249999999999997335, -29.91666666598387181, 3.031088913245538308 ) ) ;
#2349=CARTESIAN_POINT ( 'NONE',  ( -5.385316468749998364, -28.08854166632526628, 3.109213912904140287 ) ) ;
#2354=EDGE_CURVE ( 'NONE', #4014, #7159, #2739, .T. ) ;
#2357=CARTESIAN_POINT ( 'NONE',  ( -5.385316468750000141, -28.10937499965860198, 0.000000000000000000 ) ) ;
#2366=CARTESIAN_POINT ( 'NONE',  ( -5.250000000000000000, -27.43749999931720396, 0.000000000000000000 ) ) ;
#2373=CARTESIAN_POINT ( 'NONE',  ( -2.692658234375000514, -27.86979166632526628, -4.663820869356205989 ) ) ;
#2375=DIRECTION ( 'NONE',  ( 0.000000000000000000, 0.000000000000000000, -1.000000000000000000 ) ) ;
#2377=CARTESIAN_POINT ( 'NONE',  ( 1.142306659890740623E-15, -28.51562499965860198, 6.218427825808274356 ) ) ;
#2379=EDGE_LOOP ( 'NONE', ( #3605, #5087, #281, #6152 ) ) ;
#2383=CARTESIAN_POINT ( 'NONE',  ( 2.624999999999998668, -27.58333333333333570, -4.546633369868303021 ) ) ;
#2397=CARTESIAN_POINT ( 'NONE',  ( -5.385316468749998364, -27.33854166632526628, 3.109213912904140287 ) ) ;
#2400=CARTESIAN_POINT ( 'NONE',  ( -2.692658234375000514, -27.40104166632526628, -4.663820869356205989 ) ) ;
#2401=ORIENTED_EDGE ( 'NONE', *, *, #8673, .F. ) ;
#2402=CARTESIAN_POINT ( 'NONE',  ( -6.972266317189433020E-16, -28.49999999931720041, -5.249999999999999112 ) ) ;
#2404=CARTESIAN_POINT ( 'NONE',  ( 5.385316468750001029, -28.25520833299193413, 3.109213912904135846 ) ) ;
#2407=CARTESIAN_POINT ( 'NONE',  ( 5.385316468750001029, -27.22395833299193413, 3.109213912904134958 ) ) ;
#2411=CARTESIAN_POINT ( 'NONE',  ( -3.712013335537174572E-16, -28.49999999931720396, -6.062177826491070398 ) ) ;
#2414=EDGE_CURVE ( 'NONE', #4395, #3979, #8542, .T. ) ;
#2415=CARTESIAN_POINT ( 'NONE',  ( 5.250000000000000888, -29.58333333265053611, 3.031088913245533423 ) ) ;
#2418=CARTESIAN_POINT ( 'NONE',  ( -5.385316468750001029, -27.84895833299193413, -3.109213912904136734 ) ) ;
#2422=CARTESIAN_POINT ( 'NONE',  ( 5.385316468750000141, -28.70312499965860198, -6.595110575850215044E-16 ) ) ;
#2424=VECTOR ( 'NONE', #9129, 1000.000000000000000 ) ;
#2430=AXIS2_PLACEMENT_3D ( 'NONE', #6224, #8867, #5333 ) ;
#2431=VERTEX_POINT ( 'NONE', #7805 ) ;
#2433=CARTESIAN_POINT ( 'NONE',  ( -5.250000000000000000, -27.77083333333333215, -3.031088913245534755 ) ) ;
#2434=VERTEX_POINT ( 'NONE', #635 ) ;
#2438=CARTESIAN_POINT ( 'NONE',  ( -2.624999999999996891, -27.70833333333333215, 4.546633369868304797 ) ) ;
#2445=EDGE_CURVE ( 'NONE', #7820, #4395, #9183, .T. ) ;
#2448=CARTESIAN_POINT ( 'NONE',  ( 5.385316468750000141, -29.23437499965859843, -6.595110575850215044E-16 ) ) ;
#2451=CARTESIAN_POINT ( 'NONE',  ( 1.142306659890740623E-15, -27.54687499965860198, 6.218427825808274356 ) ) ;
#2455=CARTESIAN_POINT ( 'NONE',  ( 5.385316468750000141, -28.48437499965860198, -6.595110575850215044E-16 ) ) ;
#2461=CARTESIAN_POINT ( 'NONE',  ( 1.113604000661152470E-15, -27.37499999931720041, 6.062177826491070398 ) ) ;
#2462=CARTESIAN_POINT ( 'NONE',  ( -5.249999999999997335, -27.66666666598386826, 3.031088913245538308 ) ) ;
#2465=EDGE_LOOP ( 'NONE', ( #1482, #323, #2987, #1925 ) ) ;
#2467=CARTESIAN_POINT ( 'NONE',  ( 2.692658234374998738, -28.66145833299193413, -4.663820869356206877 ) ) ;
#2470=VERTEX_POINT ( 'NONE', #1422 ) ;
#2471=CARTESIAN_POINT ( 'NONE',  ( -2.692658234374996518, -28.28645833299193413, 4.663820869356208654 ) ) ;
#2475=EDGE_CURVE ( 'NONE', #27, #610, #9074, .T. ) ;
#2492=DIRECTION ( 'NONE',  ( 0.000000000000000000, -1.000000000000000000, 0.000000000000000000 ) ) ;
#2493=CARTESIAN_POINT ( 'NONE',  ( 2.692658234375002735, -29.27604166632526983, 4.663820869356205101 ) ) ;
#2495=CARTESIAN_POINT ( 'NONE',  ( 2.692658234374998738, -28.94270833299193413, -4.663820869356206877 ) ) ;
#2500=CARTESIAN_POINT ( 'NONE',  ( -5.385316468750000141, -29.35937499965859843, 0.000000000000000000 ) ) ;
#2502=CARTESIAN_POINT ( 'NONE',  ( -2.692658234374996518, -28.28645833299193413, 4.663820869356208654 ) ) ;
#2508=AXIS2_PLACEMENT_3D ( 'NONE', #5155, #2327, #2375 ) ;
#2510=CARTESIAN_POINT ( 'NONE',  ( 0.000000000000000000, -50.00000000000000000, -2.786798956483056422 ) ) ;
#2512=CARTESIAN_POINT ( 'NONE',  ( 5.385316468750001029, -28.97395833299193413, 3.109213912904135846 ) ) ;
#2513=EDGE_CURVE ( 'NONE', #8050, #1074, #6394, .T. ) ;
#2516=CARTESIAN_POINT ( 'NONE',  ( -5.385316468750000141, -28.57812499965860198, 0.000000000000000000 ) ) ;
#2518=ORIENTED_EDGE ( 'NONE', *, *, #6208, .F. ) ;
#2524=VERTEX_POINT ( 'NONE', #5697 ) ;
#2526=CARTESIAN_POINT ( 'NONE',  ( 1.113604000661152470E-15, -28.93749999999999645, 6.062177826491070398 ) ) ;
#2527=VERTEX_POINT ( 'NONE', #2169 ) ;
#2532=DIRECTION ( 'NONE',  ( -1.000000000000000000, 0.000000000000000000, -0.000000000000000000 ) ) ;
#2534=CARTESIAN_POINT ( 'NONE',  ( -5.249999999999997335, -29.97916666666666430, 3.031088913245538308 ) ) ;
#2535=VECTOR ( 'NONE', #1362, 1000.000000000000000 ) ;
#2542=CARTESIAN_POINT ( 'NONE',  ( -2.692658234375000514, -28.40104166632526628, -4.663820869356205989 ) ) ;
#2545=CARTESIAN_POINT ( 'NONE',  ( 2.692658234375002735, -29.27604166632526983, 4.663820869356205101 ) ) ;
#2553=CARTESIAN_POINT ( 'NONE',  ( -2.692658234375000514, -29.15104166632526983, -4.663820869356205989 ) ) ;
#2555=CIRCLE ( 'NONE', #5803, 6.250000000000000000 ) ;
#2556=CARTESIAN_POINT ( 'NONE',  ( -5.385316468749998364, -28.55729166632527338, 3.109213912904140287 ) ) ;
#2567=CARTESIAN_POINT ( 'NONE',  ( -5.385316468750000141, -29.82812499965859843, 0.000000000000000000 ) ) ;
#2568=EDGE_CURVE ( 'NONE', #6698, #2524, #6575, .T. ) ;
#2570=CARTESIAN_POINT ( 'NONE',  ( -5.249999999999999112, -29.52083333333333215, -3.031088913245534755 ) ) ;
#2571=CARTESIAN_POINT ( 'NONE',  ( 1.142306659890740623E-15, -28.76562499965860553, 6.218427825808274356 ) ) ;
#2572=EDGE_CURVE ( 'NONE', #8745, #2851, #7536, .T. ) ;
#2575=DIRECTION ( 'NONE',  ( 0.000000000000000000, 0.000000000000000000, -1.000000000000000000 ) ) ;
#2578=CARTESIAN_POINT ( 'NONE',  ( 1.113604000661152470E-15, -28.18750000000000000, 6.062177826491070398 ) ) ;
#2580=ORIENTED_EDGE ( 'NONE', *, *, #4211, .F. ) ;
#2592=CARTESIAN_POINT ( 'NONE',  ( 1.406733260263395735, -27.92633545031536713, 5.250000000000000000 ) ) ;
#2594=CARTESIAN_POINT ( 'NONE',  ( 2.692658234374998738, -28.19270833299193413, -4.663820869356206877 ) ) ;
#2595=CARTESIAN_POINT ( 'NONE',  ( -2.692658234375000514, -29.90104166632526983, -4.663820869356205989 ) ) ;
#2598=CARTESIAN_POINT ( 'NONE',  ( 2.692658234375002735, -29.02604166632526983, 4.663820869356205101 ) ) ;
#2601=CARTESIAN_POINT ( 'NONE',  ( -5.249999999999997335, -27.47916666666666430, 3.031088913245538308 ) ) ;
#2603=CARTESIAN_POINT ( 'NONE',  ( 2.692658234375002735, -29.77604166632526983, 4.663820869356205101 ) ) ;
#2607=CARTESIAN_POINT ( 'NONE',  ( -5.385316468749998364, -27.80729166632526628, 3.109213912904140287 ) ) ;
#2611=CARTESIAN_POINT ( 'NONE',  ( -5.249999999999999112, -28.45833333265053611, -3.031088913245534755 ) ) ;
#2615=EDGE_LOOP ( 'NONE', ( #3150, #8031, #999, #2255, #1305, #7191 ) ) ;
#2617=CARTESIAN_POINT ( 'NONE',  ( -5.385316468749998364, -29.05729166632526628, 3.109213912904140287 ) ) ;
#2619=CARTESIAN_POINT ( 'NONE',  ( -5.250000000000000000, -28.00000000000000000, 0.000000000000000000 ) ) ;
#2620=CARTESIAN_POINT ( 'NONE',  ( -2.692658234374996518, -29.78645833299193413, 4.663820869356208654 ) ) ;
#2624=CARTESIAN_POINT ( 'NONE',  ( 0.000000000000000000, -27.00000000000000000, 0.000000000000000000 ) ) ;
#2626=EDGE_CURVE ( 'NONE', #610, #8948, #7980, .T. ) ;
#2627=VERTEX_POINT ( 'NONE', #2402 ) ;
#2628=CARTESIAN_POINT ( 'NONE',  ( 5.250000000000000000, -28.60416666666666430, -3.031088913245536531 ) ) ;
#2639=CARTESIAN_POINT ( 'NONE',  ( 5.385316468750000141, -28.98437499965859843, -6.595110575850215044E-16 ) ) ;
#2641=CARTESIAN_POINT ( 'NONE',  ( 5.385316468749999252, -29.21354166632526628, -3.109213912904139399 ) ) ;
#2647=CARTESIAN_POINT ( 'NONE',  ( -5.385316468750001029, -29.88020833299193413, -3.109213912904136734 ) ) ;
#2648=ORIENTED_EDGE ( 'NONE', *, *, #2843, .F. ) ;
#2649=CARTESIAN_POINT ( 'NONE',  ( 1.142306659890740623E-15, -27.76562499965860198, 6.218427825808274356 ) ) ;
#2651=DIRECTION ( 'NONE',  ( 0.000000000000000000, 0.000000000000000000, -1.000000000000000000 ) ) ;
#2659=CARTESIAN_POINT ( 'NONE',  ( 5.385316468749999252, -29.43229166632526983, -3.109213912904139399 ) ) ;
#2662=FACE_OUTER_BOUND ( 'NONE', #5906, .T. ) ;
#2663=CARTESIAN_POINT ( 'NONE',  ( 5.385316468750001029, -29.72395833299193413, 3.109213912904135846 ) ) ;
#2665=CARTESIAN_POINT ( 'NONE',  ( 8.603239422292019767E-08, -29.99999999999999645, -5.249999999999998224 ) ) ;
#2669=ORIENTED_EDGE ( 'NONE', *, *, #7652, .F. ) ;
#2671=CARTESIAN_POINT ( 'NONE',  ( 5.250000000000000000, -27.85416666666666430, -3.031088913245536531 ) ) ;
#2680=CARTESIAN_POINT ( 'NONE',  ( -3.712013335537174572E-16, -29.24999999931720396, -6.062177826491070398 ) ) ;
#2682=CYLINDRICAL_SURFACE ( 'NONE', #4305, 6.250000000000000000 ) ;
#2683=CARTESIAN_POINT ( 'NONE',  ( -2.692658234374996518, -29.56770833299193413, 4.663820869356208654 ) ) ;
#2688=ORIENTED_EDGE ( 'NONE', *, *, #5430, .F. ) ;
#2692=CARTESIAN_POINT ( 'NONE',  ( -2.692658234375000514, -29.40104166632526983, -4.663820869356205989 ) ) ;
#2693=VERTEX_POINT ( 'NONE', #4445 ) ;
#2696=CYLINDRICAL_SURFACE ( 'NONE', #8459, 5.250000000000000000 ) ;
#2703=CARTESIAN_POINT ( 'NONE',  ( -5.385316468749998364, -29.30729166632526983, 3.109213912904140287 ) ) ;
#2706=CARTESIAN_POINT ( 'NONE',  ( 1.142306659890740623E-15, -29.76562499965859843, 6.218427825808274356 ) ) ;
#2715=CARTESIAN_POINT ( 'NONE',  ( -3.712013335537174572E-16, -28.31250000000000355, -6.062177826491070398 ) ) ;
#2724=CARTESIAN_POINT ( 'NONE',  ( 2.625000000000002220, -28.85416666598386826, 4.546633369868302132 ) ) ;
#2725=CARTESIAN_POINT ( 'NONE',  ( 2.692658234375002735, -29.52604166632526983, 4.663820869356205101 ) ) ;
#2727=CIRCLE ( 'NONE', #5676, 6.250000000000000000 ) ;
#2728=CARTESIAN_POINT ( 'NONE',  ( -5.250000000000000000, -27.00000000000000000, 0.000000000000000000 ) ) ;
#2732=ORIENTED_EDGE ( 'NONE', *, *, #4401, .T. ) ;
#2734=DIRECTION ( 'NONE',  ( 0.000000000000000000, 0.000000000000000000, -1.000000000000000000 ) ) ;
#2736=EDGE_CURVE ( 'NONE', #2202, #7225, #7481, .T. ) ;
#2737=CARTESIAN_POINT ( 'NONE',  ( -5.250000000000000000, -27.18749999931720396, 0.000000000000000000 ) ) ;
#2738=VECTOR ( 'NONE', #6424, 1000.000000000000000 ) ;
#2739=( BOUNDED_CURVE ( )  B_SPLINE_CURVE ( 2, ( #4311, #4990, #1379, #2038, #2835, #6439, #3439, #2123, #770 ),
 .UNSPECIFIED., .F., .F. ) 
 B_SPLINE_CURVE_WITH_KNOTS ( ( 3, 2, 2, 2, 3 ),
 ( 0.6458333333333333703, 0.6527777777777777901, 0.6666666666666666297, 0.6805555555555555802, 0.6875000000000000000 ),
 .UNSPECIFIED. ) 
 CURVE ( )  GEOMETRIC_REPRESENTATION_ITEM ( )  RATIONAL_B_SPLINE_CURVE ( ( 0.9330127018922192983, 0.9330127018922198534, 1.000000000000000000, 0.8660254037844387076, 1.000000000000000000, 0.8660254037844387076, 1.000000000000000000, 0.9330127018922194093, 0.9330127018922194093 ) ) 
 REPRESENTATION_ITEM ( '' )  );
#2742=ORIENTED_EDGE ( 'NONE', *, *, #5944, .F. ) ;
#2743=CARTESIAN_POINT ( 'NONE',  ( 5.385316468749999252, -29.68229166632527338, -3.109213912904138954 ) ) ;
#2745=DIRECTION ( 'NONE',  ( 0.000000000000000000, -1.000000000000000000, 0.000000000000000000 ) ) ;
#2750=CARTESIAN_POINT ( 'NONE',  ( -2.624999999999996891, -28.14583333265053255, 4.546633369868304797 ) ) ;
#2751=CARTESIAN_POINT ( 'NONE',  ( 0.000000000000000000, -30.00000000000000000, 0.000000000000000000 ) ) ;
#2755=CARTESIAN_POINT ( 'NONE',  ( -5.385316468750001029, -29.34895833299193413, -3.109213912904136734 ) ) ;
#2757=CARTESIAN_POINT ( 'NONE',  ( 5.250000000000000000, -30.06249999931720041, -6.429395695523604153E-16 ) ) ;
#2760=DIRECTION ( 'NONE',  ( 0.000000000000000000, -1.000000000000000000, 0.000000000000000000 ) ) ;
#2762=SURFACE_SIDE_STYLE ('',( #1881 ) ) ;
#2763=CARTESIAN_POINT ( 'NONE',  ( 2.624999999999998668, -29.83333333333333215, -4.546633369868303021 ) ) ;
#2772=CARTESIAN_POINT ( 'NONE',  ( -2.624999999999996891, -28.70833333333333215, 4.546633369868304797 ) ) ;
#2773=CARTESIAN_POINT ( 'NONE',  ( 1.113604000661152470E-15, -28.62499999931720041, 6.062177826491070398 ) ) ;
#2775=CYLINDRICAL_SURFACE ( 'NONE', #9102, 6.250000000000000000 ) ;
#2779=VERTEX_POINT ( 'NONE', #6918 ) ;
#2780=CARTESIAN_POINT ( 'NONE',  ( -5.317658234375000070, -30.14843749948790119, 0.000000000000000000 ) ) ;
#2784=CARTESIAN_POINT ( 'NONE',  ( 2.692658234375002735, -28.99479166632526983, 4.663820869356205101 ) ) ;
#2789=LINE ( 'NONE', #5040, #7330 ) ;
#2793=FACE_OUTER_BOUND ( 'NONE', #807, .T. ) ;
#2795=CARTESIAN_POINT ( 'NONE',  ( -2.624999999999996891, -28.64583333265053611, 4.546633369868304797 ) ) ;
#2799=CARTESIAN_POINT ( 'NONE',  ( -3.807688866302469071E-16, -29.89062499965859843, -6.218427825808274356 ) ) ;
#2805=CARTESIAN_POINT ( 'NONE',  ( 5.250000000000000000, -29.87500000000000000, -6.429395695523604153E-16 ) ) ;
#2816=CARTESIAN_POINT ( 'NONE',  ( -2.624999999999996891, -29.39583333265053611, 4.546633369868304797 ) ) ;
#2817=CARTESIAN_POINT ( 'NONE',  ( 2.625000000000002220, -27.60416666598386826, 4.546633369868302132 ) ) ;
#2819=CARTESIAN_POINT ( 'NONE',  ( -5.249999999999999112, -27.20833333265053611, -3.031088913245534755 ) ) ;
#2823=VERTEX_POINT ( 'NONE', #8221 ) ;
#2825=CARTESIAN_POINT ( 'NONE',  ( -2.624999999999996891, -28.89583333265053611, 4.546633369868304797 ) ) ;
#2830=CARTESIAN_POINT ( 'NONE',  ( 5.385316468749999252, -29.18229166632526983, -3.109213912904138954 ) ) ;
#2833=AXIS2_PLACEMENT_3D ( 'NONE', #2914, #5731, #2734 ) ;
#2835=CARTESIAN_POINT ( 'NONE',  ( -5.250000000000000000, -28.99999999999999645, 0.000000000000000000 ) ) ;
#2839=CARTESIAN_POINT ( 'NONE',  ( -5.249999999999999112, -28.20833333265053255, -3.031088913245534755 ) ) ;
#2841=CARTESIAN_POINT ( 'NONE',  ( -9.180150650966086169E-15, -28.62499999931720396, 5.250000000000000000 ) ) ;
#2843=EDGE_CURVE ( 'NONE', #7570, #8796, #8078, .T. ) ;
#2845=CARTESIAN_POINT ( 'NONE',  ( 5.385316468750000141, -27.48437499965860198, -6.595110575850215044E-16 ) ) ;
#2851=VERTEX_POINT ( 'NONE', #6956 ) ;
#2853=CARTESIAN_POINT ( 'NONE',  ( -5.250000000000000000, -30.00000000000000000, 0.000000000000000000 ) ) ;
#2854=EDGE_CURVE ( 'NONE', #7159, #8870, #471, .T. ) ;
#2858=CARTESIAN_POINT ( 'NONE',  ( 2.624999999999998668, -29.33333333333333215, -4.546633369868303021 ) ) ;
#2861=CARTESIAN_POINT ( 'NONE',  ( 5.250000000000000888, -28.83333333265053611, 3.031088913245532979 ) ) ;
#2862=CARTESIAN_POINT ( 'NONE',  ( 1.975475456537005874E-15, -27.62499999931720041, 5.250000000000000000 ) ) ;
#2867=ORIENTED_EDGE ( 'NONE', *, *, #546, .T. ) ;
#2871=ORIENTED_EDGE ( 'NONE', *, *, #814, .T. ) ;
#2872=CARTESIAN_POINT ( 'NONE',  ( -2.692658234375000514, -29.86979166632526983, -4.663820869356205989 ) ) ;
#2878=DIRECTION ( 'NONE',  ( 0.000000000000000000, -1.000000000000000000, 0.000000000000000000 ) ) ;
#2881=CARTESIAN_POINT ( 'NONE',  ( -2.033577675846918216E-14, -28.93750000000000000, 5.250000000000000888 ) ) ;
#2882=MECHANICAL_DESIGN_GEOMETRIC_PRESENTATION_REPRESENTATION('',(#1097),#1531);
#2889=CARTESIAN_POINT ( 'NONE',  ( -2.692658234375000514, -28.15104166632526628, -4.663820869356205989 ) ) ;
#2895=CARTESIAN_POINT ( 'NONE',  ( 5.385316468750001029, -27.47395833299193413, 3.109213912904135846 ) ) ;
#2899=ORIENTED_EDGE ( 'NONE', *, *, #1197, .T. ) ;
#2901=PLANE ( 'NONE',  #5691 ) ;
#2902=( BOUNDED_CURVE ( )  B_SPLINE_CURVE ( 2, ( #7900, #7945, #1519, #4364, #821, #863, #3712, #2407, #6537, #170, #3020, #2315, #7335, #8032, #3761, #5190, #5141, #7984, #1663, #1612, #4450, #7289, #961, #914, #6590, #4504, #8862, #3249, #4043, #4639, #8179, #7620, #3391, #2649, #1860, #2607, #1058, #1808, #3901, #7477, #6220, #1247, #9050, #8271, #6722, #4730, #354, #3346, #8956, #452, #4778, #1107, #4685, #6125, #548, #1902, #401, #1151, #2502, #6025, #6072, #4594, #4087, #8909, #8318, #7572, #9003, #1201, #6875, #5423, #503, #2556, #6922, #6176, #5471, #5283, #1948, #3947, #8227, #8130, #3206, #1758, #6774, #7432, #5326, #5376, #7522, #3994, #6827, #3298, #1287, #2119, #2784, #592, #4258, #4127, #1375, #5604, #2076, #4821, #8408, #2830, #6961, #674, #4173, #7092, #9139, #4985, #6264, #3435, #8449, #1459, #7706, #632, #4902, #9095, #5649, #3476, #5521, #2035, #7842, #5693, #8538, #6344, #3518, #2743, #765, #6303, #5563, #3607, #1418, #7753, #7665, #4306, #2872, #716, #4858, #7801, #9178, #3564, #1331, #7142, #7007, #4945, #4218 ),
 .UNSPECIFIED., .F., .F. ) 
 B_SPLINE_CURVE_WITH_KNOTS ( ( 3, 2, 2, 2, 2, 2, 2, 2, 2, 2, 2, 2, 2, 2, 2, 2, 2, 2, 2, 2, 2, 2, 2, 2, 2, 2, 2, 2, 2, 2, 2, 2, 2, 2, 2, 2, 2, 2, 2, 2, 2, 2, 2, 2, 2, 2, 2, 2, 2, 2, 2, 2, 2, 2, 2, 2, 2, 2, 2, 2, 2, 2, 2, 2, 2, 2, 2, 2, 2, 2, 2, 2, 3 ),
 ( 0.000000000000000000, 0.01388888888888888812, 0.02777777777777777624, 0.04166666666666666435, 0.05555555555555555247, 0.06944444444444444753, 0.08333333333333332871, 0.09722222222222222376, 0.1111111111111111049, 0.1250000000000000000, 0.1388888888888888951, 0.1527777777777777901, 0.1666666666666666574, 0.1805555555555555525, 0.1944444444444444475, 0.2083333333333333426, 0.2222222222222222099, 0.2361111111111111049, 0.2500000000000000000, 0.2638888888888888951, 0.2777777777777777901, 0.2916666666666666852, 0.3055555555555555802, 0.3194444444444444198, 0.3333333333333333148, 0.3472222222222222099, 0.3611111111111111049, 0.3750000000000000000, 0.3888888888888888951, 0.4027777777777777901, 0.4166666666666666852, 0.4305555555555555802, 0.4444444444444444198, 0.4583333333333333148, 0.4722222222222222099, 0.4861111111111111049, 0.5000000000000000000, 0.5138888888888888395, 0.5277777777777777901, 0.5416666666666666297, 0.5555555555555555802, 0.5694444444444444198, 0.5833333333333333703, 0.5972222222222222099, 0.6111111111111111605, 0.6250000000000000000, 0.6388888888888888395, 0.6527777777777777901, 0.6666666666666666297, 0.6805555555555555802, 0.6944444444444444198, 0.7083333333333333703, 0.7222222222222222099, 0.7361111111111111605, 0.7500000000000000000, 0.7638888888888888395, 0.7777777777777777901, 0.7916666666666666297, 0.8055555555555555802, 0.8194444444444444198, 0.8333333333333333703, 0.8472222222222222099, 0.8611111111111111605, 0.8750000000000000000, 0.8888888888888888395, 0.9027777777777777901, 0.9166666666666666297, 0.9305555555555555802, 0.9444444444444444198, 0.9583333333333333703, 0.9722222222222222099, 0.9861111111111111605, 1.000000000000000000 ),
 .UNSPECIFIED. ) 
 CURVE ( )  GEOMETRIC_REPRESENTATION_ITEM ( )  RATIONAL_B_SPLINE_CURVE ( ( 1.000000000000000000, 0.8660254037844387076, 1.000000000000000000, 0.8660254037844387076, 1.000000000000000000, 0.8660254037844387076, 1.000000000000000000, 0.8660254037844387076, 1.000000000000000000, 0.8660254037844387076, 1.000000000000000000, 0.8660254037844387076, 1.000000000000000000, 0.8660254037844387076, 1.000000000000000000, 0.8660254037844387076, 1.000000000000000000, 0.8660254037844387076, 1.000000000000000000, 0.8660254037844387076, 1.000000000000000000, 0.8660254037844387076, 1.000000000000000000, 0.8660254037844387076, 1.000000000000000000, 0.8660254037844387076, 1.000000000000000000, 0.8660254037844387076, 1.000000000000000000, 0.8660254037844387076, 1.000000000000000000, 0.8660254037844387076, 1.000000000000000000, 0.8660254037844387076, 1.000000000000000000, 0.8660254037844387076, 1.000000000000000000, 0.8660254037844387076, 1.000000000000000000, 0.8660254037844387076, 1.000000000000000000, 0.8660254037844387076, 1.000000000000000000, 0.8660254037844387076, 1.000000000000000000, 0.8660254037844387076, 1.000000000000000000, 0.8660254037844387076, 1.000000000000000000, 0.8660254037844387076, 1.000000000000000000, 0.8660254037844387076, 1.000000000000000000, 0.8660254037844387076, 1.000000000000000000, 0.8660254037844387076, 1.000000000000000000, 0.8660254037844387076, 1.000000000000000000, 0.8660254037844387076, 1.000000000000000000, 0.8660254037844387076, 1.000000000000000000, 0.8660254037844387076, 1.000000000000000000, 0.8660254037844387076, 1.000000000000000000, 0.8660254037844387076, 1.000000000000000000, 0.8660254037844387076, 1.000000000000000000, 0.8660254037844387076, 1.000000000000000000, 0.8660254037844387076, 1.000000000000000000, 0.8660254037844387076, 1.000000000000000000, 0.8660254037844387076, 1.000000000000000000, 0.8660254037844387076, 1.000000000000000000, 0.8660254037844387076, 1.000000000000000000, 0.8660254037844387076, 1.000000000000000000, 0.8660254037844387076, 1.000000000000000000, 0.8660254037844387076, 1.000000000000000000, 0.8660254037844387076, 1.000000000000000000, 0.8660254037844387076, 1.000000000000000000, 0.8660254037844387076, 1.000000000000000000, 0.8660254037844387076, 1.000000000000000000, 0.8660254037844387076, 1.000000000000000000, 0.8660254037844387076, 1.000000000000000000, 0.8660254037844387076, 1.000000000000000000, 0.8660254037844387076, 1.000000000000000000, 0.8660254037844387076, 1.000000000000000000, 0.8660254037844387076, 1.000000000000000000, 0.8660254037844387076, 1.000000000000000000, 0.8660254037844387076, 1.000000000000000000, 0.8660254037844387076, 1.000000000000000000, 0.8660254037844387076, 1.000000000000000000, 0.8660254037844387076, 1.000000000000000000, 0.8660254037844387076, 1.000000000000000000, 0.8660254037844387076, 1.000000000000000000, 0.8660254037844387076, 1.000000000000000000, 0.8660254037844387076, 1.000000000000000000, 0.8660254037844387076, 1.000000000000000000, 0.8660254037844387076, 1.000000000000000000, 0.8660254037844387076, 1.000000000000000000, 0.8660254037844387076, 1.000000000000000000, 0.8660254037844387076, 1.000000000000000000, 0.8660254037844387076, 1.000000000000000000, 0.8660254037844387076, 1.000000000000000000, 0.8660254037844387076, 1.000000000000000000, 0.8660254037844387076, 1.000000000000000000 ) ) 
 REPRESENTATION_ITEM ( '' )  );
#2914=CARTESIAN_POINT ( 'NONE',  ( 0.000000000000000000, -27.00000000000000000, 0.000000000000000000 ) ) ;
#2916=ORIENTED_EDGE ( 'NONE', *, *, #924, .F. ) ;
#2917=EDGE_CURVE ( 'NONE', #1598, #6037, #1326, .T. ) ;
#2919=CARTESIAN_POINT ( 'NONE',  ( 2.624999999999998668, -29.58333333333333215, -4.546633369868303021 ) ) ;
#2927=DIRECTION ( 'NONE',  ( 0.000000000000000000, -1.000000000000000000, 0.000000000000000000 ) ) ;
#2931=CARTESIAN_POINT ( 'NONE',  ( 1.142306659890740623E-15, -28.29687499965860553, 6.218427825808274356 ) ) ;
#2937=CARTESIAN_POINT ( 'NONE',  ( 1.142306659890740623E-15, -27.26562499965860553, 6.218427825808274356 ) ) ;
#2939=DIRECTION ( 'NONE',  ( 0.000000000000000000, -1.000000000000000000, 0.000000000000000000 ) ) ;
#2944=EDGE_CURVE ( 'NONE', #4857, #7379, #5220, .T. ) ;
#2951=CARTESIAN_POINT ( 'NONE',  ( -5.317658234375000070, -27.14843749948790119, 0.000000000000000000 ) ) ;
#2961=CARTESIAN_POINT ( 'NONE',  ( 1.406733260263385521, -29.67633545031537423, 5.250000000000006217 ) ) ;
#2962=CARTESIAN_POINT ( 'NONE',  ( -2.692658234375000514, -27.40104166632526628, -4.663820869356205989 ) ) ;
#2966=ORIENTED_EDGE ( 'NONE', *, *, #7789, .F. ) ;
#2978=CARTESIAN_POINT ( 'NONE',  ( 1.406733260263393293, -27.57366454968463643, -5.250000000000000000 ) ) ;
#2981=CARTESIAN_POINT ( 'NONE',  ( -2.033577675846918216E-14, -29.12499999931720751, 5.250000000000000888 ) ) ;
#2984=CARTESIAN_POINT ( 'NONE',  ( 2.692658234375002735, -28.74479166632526628, 4.663820869356205101 ) ) ;
#2987=ORIENTED_EDGE ( 'NONE', *, *, #4754, .T. ) ;
#2988=CARTESIAN_POINT ( 'NONE',  ( 5.385316468749999252, -27.68229166632526272, -3.109213912904139399 ) ) ;
#3005=CARTESIAN_POINT ( 'NONE',  ( 1.406733260263395735, -27.17633545031536713, 5.250000000000000000 ) ) ;
#3010=CARTESIAN_POINT ( 'NONE',  ( 5.385316468750001029, -27.25520833299193413, 3.109213912904134958 ) ) ;
#3012=CARTESIAN_POINT ( 'NONE',  ( 0.000000000000000000, -29.87813065659485190, 0.000000000000000000 ) ) ;
#3015=EDGE_CURVE ( 'NONE', #8099, #6175, #4626, .T. ) ;
#3016=CARTESIAN_POINT ( 'NONE',  ( 5.385316468750000141, -27.98437499965860198, -6.595110575850215044E-16 ) ) ;
#3020=CARTESIAN_POINT ( 'NONE',  ( -2.692658234374996518, -27.28645833299193413, 4.663820869356208654 ) ) ;
#3023=FACE_OUTER_BOUND ( 'NONE', #2465, .T. ) ;
#3025=AXIS2_PLACEMENT_3D ( 'NONE', #3354, #599, #1958 ) ;
#3027=CARTESIAN_POINT ( 'NONE',  ( 2.624999999999998668, -28.27083333265053255, -4.546633369868303021 ) ) ;
#3030=CARTESIAN_POINT ( 'NONE',  ( 1.975475456537005874E-15, -29.62499999931719685, 5.250000000000000000 ) ) ;
#3034=CARTESIAN_POINT ( 'NONE',  ( 2.692658234375002735, -27.74479166632526628, 4.663820869356205101 ) ) ;
#3037=CARTESIAN_POINT ( 'NONE',  ( -1.406733260263397289, -28.44866454968463998, 5.249999999999997335 ) ) ;
#3041=ORIENTED_EDGE ( 'NONE', *, *, #1120, .F. ) ;
#3049=EDGE_CURVE ( 'NONE', #3470, #8050, #6836, .T. ) ;
#3050=CARTESIAN_POINT ( 'NONE',  ( -2.624999999999996891, -29.89583333265053611, 4.546633369868304797 ) ) ;
#3054=CARTESIAN_POINT ( 'NONE',  ( 1.406733260263398400, -28.01116454900182973, -5.249999999999997335 ) ) ;
#3058=CARTESIAN_POINT ( 'NONE',  ( -2.033577675846918216E-14, -29.68750000000000355, 5.250000000000000888 ) ) ;
#3060=CARTESIAN_POINT ( 'NONE',  ( 2.692658234374998738, -27.94270833299193413, -4.663820869356206877 ) ) ;
#3067=CARTESIAN_POINT ( 'NONE',  ( 2.692658234374998738, -27.94270833299193413, -4.663820869356206877 ) ) ;
#3073=CARTESIAN_POINT ( 'NONE',  ( -2.625000000000000444, -27.72916666598386826, -4.546633369868303021 ) ) ;
#3074=CARTESIAN_POINT ( 'NONE',  ( 5.250000000000000000, -27.62500000000000000, -6.429395695523604153E-16 ) ) ;
#3078=CARTESIAN_POINT ( 'NONE',  ( 5.385316468749999252, -28.68229166632526983, -3.109213912904139399 ) ) ;
#3082=CARTESIAN_POINT ( 'NONE',  ( -5.249999999999997335, -27.22916666666666430, 3.031088913245538308 ) ) ;
#3087=( BOUNDED_CURVE ( )  B_SPLINE_CURVE ( 2, ( #6880, #1955, #2171, #6308, #4265, #1515, #31, #3571, #2881 ),
 .UNSPECIFIED., .F., .T. ) 
 B_SPLINE_CURVE_WITH_KNOTS ( ( 3, 2, 2, 2, 3 ),
 ( 0.6041666666666667407, 0.6111111111111111605, 0.6250000000000000000, 0.6388888888888888395, 0.6458333333333333703 ),
 .UNSPECIFIED. ) 
 CURVE ( )  GEOMETRIC_REPRESENTATION_ITEM ( )  RATIONAL_B_SPLINE_CURVE ( ( 0.9330127018922192983, 0.9330127018922198534, 1.000000000000000000, 0.8660254037844387076, 1.000000000000000000, 0.8660254037844387076, 1.000000000000000000, 0.9330127018922187432, 0.9330127018922192983 ) ) 
 REPRESENTATION_ITEM ( '' )  );
#3088=CARTESIAN_POINT ( 'NONE',  ( -5.250000000000000000, -27.50000000000000000, 0.000000000000000000 ) ) ;
#3091=CARTESIAN_POINT ( 'NONE',  ( 2.161402558328724325E-14, -28.56250000000000000, -5.250000000000000000 ) ) ;
#3094=COLOUR_RGB ( '',0.8941176470588234615, 0.8941176470588234615, 0.8941176470588234615 ) ;
#3104=CARTESIAN_POINT ( 'NONE',  ( 2.692658234375002735, -27.77604166632526628, 4.663820869356205101 ) ) ;
#3107=CARTESIAN_POINT ( 'NONE',  ( -5.249999999999997335, -27.91666666598387181, 3.031088913245538308 ) ) ;
#3109=CARTESIAN_POINT ( 'NONE',  ( 5.385316468750000141, -27.73437499965860198, -6.595110575850215044E-16 ) ) ;
#3112=AXIS2_PLACEMENT_3D ( 'NONE', #823, #5047, #7062 ) ;
#3113=CARTESIAN_POINT ( 'NONE',  ( 2.625000000000002220, -28.85416666598386826, 4.546633369868302132 ) ) ;
#3117=CARTESIAN_POINT ( 'NONE',  ( 5.250000000000000000, -27.54166666598386470, -3.031088913245536531 ) ) ;
#3124=CARTESIAN_POINT ( 'NONE',  ( -5.385316468749998364, -28.55729166632527338, 3.109213912904140287 ) ) ;
#3129=CARTESIAN_POINT ( 'NONE',  ( 2.692658234375002735, -28.24479166632526628, 4.663820869356205101 ) ) ;
#3138=CARTESIAN_POINT ( 'NONE',  ( -3.712013335537174572E-16, -27.56250000000000000, -6.062177826491070398 ) ) ;
#3144=CARTESIAN_POINT ( 'NONE',  ( -5.250000000000000000, -30.09374999965860198, 0.000000000000000000 ) ) ;
#3147=CARTESIAN_POINT ( 'NONE',  ( 1.975475456537005874E-15, -27.68749999999999289, 5.249999999999999112 ) ) ;
#3150=ORIENTED_EDGE ( 'NONE', *, *, #4703, .F. ) ;
#3151=CARTESIAN_POINT ( 'NONE',  ( 0.000000000000000000, -30.00000000000000000, 0.000000000000000000 ) ) ;
#3152=CARTESIAN_POINT ( 'NONE',  ( -5.385316468750000141, -28.10937499965860198, 0.000000000000000000 ) ) ;
#3154=CARTESIAN_POINT ( 'NONE',  ( 5.385316468750001029, -27.50520833299193768, 3.109213912904135846 ) ) ;
#3156=CARTESIAN_POINT ( 'NONE',  ( 5.250000000000000000, -29.87500000000000000, -6.429395695523604153E-16 ) ) ;
#3158=CARTESIAN_POINT ( 'NONE',  ( -3.807688866302469071E-16, -28.42187499965859843, -6.218427825808274356 ) ) ;
#3164=CARTESIAN_POINT ( 'NONE',  ( 5.250000000000000000, -28.04166666598386826, -3.031088913245536531 ) ) ;
#3170=CARTESIAN_POINT ( 'NONE',  ( 5.385316468749999252, -28.18229166632526628, -3.109213912904139399 ) ) ;
#3173=CARTESIAN_POINT ( 'NONE',  ( -2.692658234375000514, -28.11979166632526628, -4.663820869356205989 ) ) ;
#3181=ORIENTED_EDGE ( 'NONE', *, *, #3839, .F. ) ;
#3182=CARTESIAN_POINT ( 'NONE',  ( 2.625000000000002220, -27.16666666666666430, 4.546633369868302132 ) ) ;
#3194=CARTESIAN_POINT ( 'NONE',  ( 5.250000000000000888, -27.89583333333332860, 3.031088913245533423 ) ) ;
#3195=CARTESIAN_POINT ( 'NONE',  ( -5.385316468749998364, -29.33854166632526983, 3.109213912904140287 ) ) ;
#3198=CARTESIAN_POINT ( 'NONE',  ( 2.692658234374998738, -29.19270833299193413, -4.663820869356206877 ) ) ;
#3203=CARTESIAN_POINT ( 'NONE',  ( 2.692658234375002735, -27.27604166632526628, 4.663820869356205101 ) ) ;
#3206=CARTESIAN_POINT ( 'NONE',  ( 2.692658234375002735, -28.74479166632526628, 4.663820869356205101 ) ) ;
#3214=CARTESIAN_POINT ( 'NONE',  ( -2.692658234374996518, -29.28645833299193413, 4.663820869356208654 ) ) ;
#3216=CARTESIAN_POINT ( 'NONE',  ( 0.000000000000000000, -27.00000000000000000, 0.000000000000000000 ) ) ;
#3218=CARTESIAN_POINT ( 'NONE',  ( -2.692658234375000514, -28.36979166632526628, -4.663820869356205989 ) ) ;
#3220=VERTEX_POINT ( 'NONE', #3147 ) ;
#3224=VERTEX_POINT ( 'NONE', #5919 ) ;
#3225=CARTESIAN_POINT ( 'NONE',  ( -5.250000000000000000, -27.00000000000000000, 0.000000000000000000 ) ) ;
#3226=VERTEX_POINT ( 'NONE', #8762 ) ;
#3231=DIRECTION ( 'NONE',  ( 0.000000000000000000, 0.000000000000000000, -1.000000000000000000 ) ) ;
#3234=CARTESIAN_POINT ( 'NONE',  ( -2.033577675846918216E-14, -29.37499999931720396, 5.250000000000000888 ) ) ;
#3236=ORIENTED_EDGE ( 'NONE', *, *, #2414, .T. ) ;
#3238=CARTESIAN_POINT ( 'NONE',  ( 2.692658234375002735, -28.27604166632526628, 4.663820869356205101 ) ) ;
#3239=CARTESIAN_POINT ( 'NONE',  ( -2.692658234374996518, -29.56770833299193413, 4.663820869356208654 ) ) ;
#3241=CARTESIAN_POINT ( 'NONE',  ( -3.807688866302469071E-16, -29.92187499965859843, -6.218427825808274356 ) ) ;
#3243=VERTEX_POINT ( 'NONE', #3234 ) ;
#3246=CARTESIAN_POINT ( 'NONE',  ( -2.692658234374996518, -29.06770833299193413, 4.663820869356208654 ) ) ;
#3249=CARTESIAN_POINT ( 'NONE',  ( -3.807688866302469071E-16, -27.64062499965859843, -6.218427825808274356 ) ) ;
#3252=( BOUNDED_CURVE ( )  B_SPLINE_CURVE ( 2, ( #6312, #5045, #1384, #3487, #9106, #4229, #6271, #7152, #7015 ),
 .UNSPECIFIED., .F., .F. ) 
 B_SPLINE_CURVE_WITH_KNOTS ( ( 3, 2, 2, 2, 3 ),
 ( 0.1875000000000000000, 0.1944444444444444475, 0.2083333333333333426, 0.2222222222222222099, 0.2291666666666666574 ),
 .UNSPECIFIED. ) 
 CURVE ( )  GEOMETRIC_REPRESENTATION_ITEM ( )  RATIONAL_B_SPLINE_CURVE ( ( 0.9330127018922194093, 0.9330127018922194093, 1.000000000000000000, 0.8660254037844387076, 1.000000000000000000, 0.8660254037844387076, 1.000000000000000000, 0.9330127018922194093, 0.9330127018922194093 ) ) 
 REPRESENTATION_ITEM ( '' )  );
#3253=CARTESIAN_POINT ( 'NONE',  ( 0.000000000000000000, -27.00000000000000000, 0.000000000000000000 ) ) ;
#3254=CARTESIAN_POINT ( 'NONE',  ( 2.624999999999998668, -27.33333333333333570, -4.546633369868303021 ) ) ;
#3260=CARTESIAN_POINT ( 'NONE',  ( 0.000000000000000000, -27.00000000000000000, -5.250000000000000000 ) ) ;
#3261=CARTESIAN_POINT ( 'NONE',  ( -5.385316468750001029, -28.59895833299193413, -3.109213912904136734 ) ) ;
#3270=CARTESIAN_POINT ( 'NONE',  ( -2.624999999999996891, -28.95833333333333215, 4.546633369868304797 ) ) ;
#3271=ORIENTED_EDGE ( 'NONE', *, *, #6896, .F. ) ;
#3275=PLANE ( 'NONE',  #7022 ) ;
#3285=CARTESIAN_POINT ( 'NONE',  ( 2.625000000000002220, -27.91666666666666430, 4.546633369868302132 ) ) ;
#3286=CARTESIAN_POINT ( 'NONE',  ( 5.385316468750000141, -29.48437499965859843, -6.595110575850215044E-16 ) ) ;
#3287=CARTESIAN_POINT ( 'NONE',  ( 5.385316468749999252, -29.71354166632527338, -3.109213912904138954 ) ) ;
#3289=CARTESIAN_POINT ( 'NONE',  ( 1.142306659890740623E-15, -29.54687499965859843, 6.218427825808274356 ) ) ;
#3291=ORIENTED_EDGE ( 'NONE', *, *, #5944, .T. ) ;
#3295=CARTESIAN_POINT ( 'NONE',  ( -2.692658234375000514, -29.65104166632526983, -4.663820869356205989 ) ) ;
#3298=CARTESIAN_POINT ( 'NONE',  ( 5.385316468749999252, -28.93229166632526983, -3.109213912904138954 ) ) ;
#3300=CARTESIAN_POINT ( 'NONE',  ( -5.250000000000000000, -27.18749999931720396, 0.000000000000000000 ) ) ;
#3306=CARTESIAN_POINT ( 'NONE',  ( -5.385316468749998364, -30.05729166632526628, 3.109213912904140287 ) ) ;
#3310=CARTESIAN_POINT ( 'NONE',  ( 5.385316468750001029, -28.72395833299193413, 3.109213912904135846 ) ) ;
#3317=ORIENTED_EDGE ( 'NONE', *, *, #435, .T. ) ;
#3318=( NAMED_UNIT ( * ) PLANE_ANGLE_UNIT ( ) SI_UNIT ( $, .RADIAN. ) );
#3319=CARTESIAN_POINT ( 'NONE',  ( -2.624999999999996891, -28.45833333333333215, 4.546633369868304797 ) ) ;
#3332=( BOUNDED_CURVE ( )  B_SPLINE_CURVE ( 2, ( #7928, #3054, #3602, #7136, #5074, #6427, #7271, #1595, #4486 ),
 .UNSPECIFIED., .F., .F. ) 
 B_SPLINE_CURVE_WITH_KNOTS ( ( 3, 2, 2, 2, 3 ),
 ( 0.2708333333333333703, 0.2777777777777777901, 0.2916666666666666852, 0.3055555555555555802, 0.3125000000000000000 ),
 .UNSPECIFIED. ) 
 CURVE ( )  GEOMETRIC_REPRESENTATION_ITEM ( )  RATIONAL_B_SPLINE_CURVE ( ( 0.9330127018922194093, 0.9330127018922196314, 1.000000000000000000, 0.8660254037844387076, 1.000000000000000000, 0.8660254037844387076, 1.000000000000000000, 0.9330127018922194093, 0.9330127018922194093 ) ) 
 REPRESENTATION_ITEM ( '' )  );
#3333=FACE_BOUND ( 'NONE', #830, .T. ) ;
#3334=CARTESIAN_POINT ( 'NONE',  ( 5.385316468749999252, -28.21354166632526628, -3.109213912904138954 ) ) ;
#3338=CARTESIAN_POINT ( 'NONE',  ( 1.142306659890740623E-15, -30.04687499965860198, 6.218427825808274356 ) ) ;
#3342=CARTESIAN_POINT ( 'NONE',  ( 5.250000000000000000, -28.37500000000000000, -6.429395695523604153E-16 ) ) ;
#3344=CARTESIAN_POINT ( 'NONE',  ( -5.385316468749998364, -29.83854166632526628, 3.109213912904140287 ) ) ;
#3345=EDGE_LOOP ( 'NONE', ( #3041, #3724, #5877, #2966 ) ) ;
#3346=CARTESIAN_POINT ( 'NONE',  ( -5.385316468749998364, -28.05729166632526272, 3.109213912904140287 ) ) ;
#3350=CARTESIAN_POINT ( 'NONE',  ( 0.000000000000000000, -27.00000000000000000, 0.000000000000000000 ) ) ;
#3354=CARTESIAN_POINT ( 'NONE',  ( 0.000000000000000000, -29.87813065659485190, 0.000000000000000000 ) ) ;
#3356=CARTESIAN_POINT ( 'NONE',  ( 2.692658234375002735, -29.24479166632526983, 4.663820869356205101 ) ) ;
#3358=CARTESIAN_POINT ( 'NONE',  ( 5.250000000000000000, -28.56249999931720396, -6.429395695523604153E-16 ) ) ;
#3359=CARTESIAN_POINT ( 'NONE',  ( 5.385316468750001029, -29.22395833299193413, 3.109213912904135846 ) ) ;
#3366=CARTESIAN_POINT ( 'NONE',  ( 2.625000000000002220, -27.91666666666666430, 4.546633369868302132 ) ) ;
#3369=FACE_OUTER_BOUND ( 'NONE', #63, .T. ) ;
#3371=CARTESIAN_POINT ( 'NONE',  ( -1.406733260263394625, -29.23883544963257464, -5.250000000000000000 ) ) ;
#3375=LINE ( 'NONE', #3507, #8155 ) ;
#3376=CARTESIAN_POINT ( 'NONE',  ( -5.385316468750000141, -29.10937499965859843, 0.000000000000000000 ) ) ;
#3377=CARTESIAN_POINT ( 'NONE',  ( -5.385316468750001029, -29.88020833299193413, -3.109213912904136734 ) ) ;
#3379=CARTESIAN_POINT ( 'NONE',  ( -5.385316468750001029, -29.13020833299193058, -3.109213912904136734 ) ) ;
#3386=CARTESIAN_POINT ( 'NONE',  ( 5.385316468750001029, -29.00520833299193413, 3.109213912904135846 ) ) ;
#3389=EDGE_CURVE ( 'NONE', #7114, #2434, #6159, .T. ) ;
#3391=CARTESIAN_POINT ( 'NONE',  ( 2.692658234375002735, -27.74479166632526628, 4.663820869356205101 ) ) ;
#3402=CARTESIAN_POINT ( 'NONE',  ( -5.385316468750001029, -29.59895833299193413, -3.109213912904136734 ) ) ;
#3404=CYLINDRICAL_SURFACE ( 'NONE', #8453, 5.250000000000000000 ) ;
#3405=CARTESIAN_POINT ( 'NONE',  ( -5.385316468750001029, -29.09895833299193058, -3.109213912904136734 ) ) ;
#3410=ORIENTED_EDGE ( 'NONE', *, *, #144, .F. ) ;
#3411=CARTESIAN_POINT ( 'NONE',  ( -5.249999999999999112, -28.72916666666666785, 3.031088913245538308 ) ) ;
#3414=CARTESIAN_POINT ( 'NONE',  ( 0.000000000000000000, -27.00000000000000000, -5.250000000000000000 ) ) ;
#3422=DIRECTION ( 'NONE',  ( 0.000000000000000000, 0.000000000000000000, -1.000000000000000000 ) ) ;
#3423=CARTESIAN_POINT ( 'NONE',  ( -5.250000000000000000, -28.93749999931720396, 0.000000000000000000 ) ) ;
#3424=CARTESIAN_POINT ( 'NONE',  ( 2.692658234374998738, -29.94270833299193413, -4.663820869356206877 ) ) ;
#3426=DIRECTION ( 'NONE',  ( 0.000000000000000000, -1.000000000000000000, 0.000000000000000000 ) ) ;
#3430=DIRECTION ( 'NONE',  ( -0.8660254037844402619, 0.4999999999999970579, -0.000000000000000000 ) ) ;
#3433=CARTESIAN_POINT ( 'NONE',  ( 5.385316468749999252, -28.96354166632526983, -3.109213912904139399 ) ) ;
#3435=CARTESIAN_POINT ( 'NONE',  ( -5.385316468750001029, -29.34895833299193413, -3.109213912904136734 ) ) ;
#3439=CARTESIAN_POINT ( 'NONE',  ( -2.625000000000000444, -29.04166666666666785, -4.546633369868303021 ) ) ;
#3440=DIRECTION ( 'NONE',  ( 0.000000000000000000, -1.000000000000000000, 0.000000000000000000 ) ) ;
#3441=CARTESIAN_POINT ( 'NONE',  ( 0.000000000000000000, -27.00000000000000000, 0.000000000000000000 ) ) ;
#3448=CARTESIAN_POINT ( 'NONE',  ( -5.385316468749998364, -29.55729166632526983, 3.109213912904140287 ) ) ;
#3452=CARTESIAN_POINT ( 'NONE',  ( 5.250000000000000888, -28.14583333333333215, 3.031088913245532979 ) ) ;
#3459=VECTOR ( 'NONE', #3985, 1000.000000000000000 ) ;
#3463=CARTESIAN_POINT ( 'NONE',  ( -2.625000000000000444, -28.72916666598386826, -4.546633369868303021 ) ) ;
#3469=AXIS2_PLACEMENT_3D ( 'NONE', #5264, #6756, #3231 ) ;
#3470=VERTEX_POINT ( 'NONE', #3535 ) ;
#3476=CARTESIAN_POINT ( 'NONE',  ( 1.142306659890740623E-15, -29.51562499965859487, 6.218427825808274356 ) ) ;
#3480=VECTOR ( 'NONE', #68, 1000.000000000000000 ) ;
#3481=DIRECTION ( 'NONE',  ( 0.000000000000000000, -1.000000000000000000, 0.000000000000000000 ) ) ;
#3487=CARTESIAN_POINT ( 'NONE',  ( 5.249999999999999112, -27.79166666598386826, -3.031088913245536975 ) ) ;
#3490=CARTESIAN_POINT ( 'NONE',  ( -2.692658234375000514, -29.36979166632526983, -4.663820869356205989 ) ) ;
#3496=CARTESIAN_POINT ( 'NONE',  ( 5.250000000000000000, -29.35416666666666430, -3.031088913245536531 ) ) ;
#3507=CARTESIAN_POINT ( 'NONE',  ( 6.429395695523604153E-16, -27.00000000000000000, 5.250000000000000000 ) ) ;
#3508=CARTESIAN_POINT ( 'NONE',  ( 2.625000000000002220, -29.85416666598387181, 4.546633369868302132 ) ) ;
#3509=CYLINDRICAL_SURFACE ( 'NONE', #7625, 5.250000000000000000 ) ;
#3514=ORIENTED_EDGE ( 'NONE', *, *, #6799, .F. ) ;
#3518=CARTESIAN_POINT ( 'NONE',  ( 2.692658234374998738, -29.66145833299193413, -4.663820869356206877 ) ) ;
#3521=ORIENTED_EDGE ( 'NONE', *, *, #2354, .F. ) ;
#3525=CYLINDRICAL_SURFACE ( 'NONE', #3732, 5.250000000000000000 ) ;
#3527=FACE_OUTER_BOUND ( 'NONE', #348, .T. ) ;
#3529=CARTESIAN_POINT ( 'NONE',  ( 1.975475456537005874E-15, -28.12499999931720041, 5.250000000000000000 ) ) ;
#3530=DIRECTION ( 'NONE',  ( -0.000000000000000000, 1.000000000000000000, -0.000000000000000000 ) ) ;
#3532=CARTESIAN_POINT ( 'NONE',  ( 1.975475456537005874E-15, -29.43750000000000000, 5.249999999999999112 ) ) ;
#3533=CARTESIAN_POINT ( 'NONE',  ( 5.385316468749999252, -29.68229166632526983, -3.109213912904139399 ) ) ;
#3535=CARTESIAN_POINT ( 'NONE',  ( 0.000000000000000000, -27.00000000000000000, -5.250000000000000000 ) ) ;
#3539=CARTESIAN_POINT ( 'NONE',  ( 2.624999999999998668, -29.58333333333333215, -4.546633369868303021 ) ) ;
#3543=DIRECTION ( 'NONE',  ( 0.000000000000000000, -1.000000000000000000, 0.000000000000000000 ) ) ;
#3551=CARTESIAN_POINT ( 'NONE',  ( -2.624999999999996891, -28.64583333265053611, 4.546633369868304797 ) ) ;
#3552=CARTESIAN_POINT ( 'NONE',  ( 5.250000000000000888, -27.58333333265053611, 3.031088913245533423 ) ) ;
#3555=DIRECTION ( 'NONE',  ( 1.000000000000000000, 0.000000000000000000, 0.000000000000000000 ) ) ;
#3557=ORIENTED_EDGE ( 'NONE', *, *, #5300, .F. ) ;
#3564=CARTESIAN_POINT ( 'NONE',  ( 5.385316468750001029, -29.97395833299194123, 3.109213912904134958 ) ) ;
#3568=ORIENTED_EDGE ( 'NONE', *, *, #1863, .T. ) ;
#3571=CARTESIAN_POINT ( 'NONE',  ( 1.406733260263385521, -28.92633545031537068, 5.250000000000006217 ) ) ;
#3573=DIRECTION ( 'NONE',  ( 1.000000000000000000, 0.000000000000000000, 0.000000000000000000 ) ) ;
#3578=CARTESIAN_POINT ( 'NONE',  ( -2.692658234374996518, -28.31770833299193413, 4.663820869356208654 ) ) ;
#3584=CARTESIAN_POINT ( 'NONE',  ( 5.250000000000000888, -29.14583333333333925, 3.031088913245532979 ) ) ;
#3586=CARTESIAN_POINT ( 'NONE',  ( 1.142306659890740623E-15, -27.51562499965859843, 6.218427825808274356 ) ) ;
#3590=FACE_OUTER_BOUND ( 'NONE', #6790, .T. ) ;
#3595=( BOUNDED_CURVE ( )  B_SPLINE_CURVE ( 2, ( #58, #5594, #7128, #14, #751, #3552, #2817, #9168, #2862 ),
 .UNSPECIFIED., .F., .T. ) 
 B_SPLINE_CURVE_WITH_KNOTS ( ( 3, 2, 2, 2, 3 ),
 ( 0.1041666666666666713, 0.1111111111111111049, 0.1250000000000000000, 0.1388888888888888951, 0.1458333333333333426 ),
 .UNSPECIFIED. ) 
 CURVE ( )  GEOMETRIC_REPRESENTATION_ITEM ( )  RATIONAL_B_SPLINE_CURVE ( ( 0.9330127018922194093, 0.9330127018922194093, 1.000000000000000000, 0.8660254037844387076, 1.000000000000000000, 0.8660254037844387076, 1.000000000000000000, 0.9330127018922194093, 0.9330127018922194093 ) ) 
 REPRESENTATION_ITEM ( '' )  );
#3601=ORIENTED_EDGE ( 'NONE', *, *, #7269, .F. ) ;
#3602=CARTESIAN_POINT ( 'NONE',  ( 2.624999999999998668, -28.02083333265053255, -4.546633369868303021 ) ) ;
#3603=CARTESIAN_POINT ( 'NONE',  ( 5.250000000000000888, -29.14583333333333925, 3.031088913245533423 ) ) ;
#3605=ORIENTED_EDGE ( 'NONE', *, *, #2128, .F. ) ;
#3607=CARTESIAN_POINT ( 'NONE',  ( 1.142306659890740623E-15, -29.76562499965859843, 6.218427825808274356 ) ) ;
#3612=EDGE_LOOP ( 'NONE', ( #1079, #1555, #5444, #1413 ) ) ;
#3617=AXIS2_PLACEMENT_3D ( 'NONE', #7120, #3543, #7687 ) ;
#3621=ADVANCED_FACE ( 'NONE', ( #5101 ), #5335, .F. ) ;
#3624=( BOUNDED_CURVE ( )  B_SPLINE_CURVE ( 2, ( #3529, #7014, #2750, #8375, #2130, #2839, #6971, #5571, #9059 ),
 .UNSPECIFIED., .F., .T. ) 
 B_SPLINE_CURVE_WITH_KNOTS ( ( 3, 2, 2, 2, 3 ),
 ( 0.3125000000000000000, 0.3194444444444444198, 0.3333333333333333148, 0.3472222222222222099, 0.3541666666666666852 ),
 .UNSPECIFIED. ) 
 CURVE ( )  GEOMETRIC_REPRESENTATION_ITEM ( )  RATIONAL_B_SPLINE_CURVE ( ( 0.9330127018922194093, 0.9330127018922194093, 1.000000000000000000, 0.8660254037844387076, 1.000000000000000000, 0.8660254037844387076, 1.000000000000000000, 0.9330127018922190762, 0.9330127018922194093 ) ) 
 REPRESENTATION_ITEM ( '' )  );
#3625=CARTESIAN_POINT ( 'NONE',  ( -5.385316468750000141, -27.85937499965860198, 0.000000000000000000 ) ) ;
#3631=CARTESIAN_POINT ( 'NONE',  ( 1.142306659890740623E-15, -27.51562499965859843, 6.218427825808274356 ) ) ;
#3632=ORIENTED_EDGE ( 'NONE', *, *, #8113, .T. ) ;
#3633=CARTESIAN_POINT ( 'NONE',  ( -5.385316468750001029, -27.34895833299193768, -3.109213912904136734 ) ) ;
#3635=ADVANCED_BREP_SHAPE_REPRESENTATION ( '', ( #5214, #888 ), #6484 ) ;
#3641=CARTESIAN_POINT ( 'NONE',  ( 5.250000000000000000, -30.06249999931720041, -6.429395695523604153E-16 ) ) ;
#3642=LINE ( 'NONE', #2951, #4509 ) ;
#3644=CARTESIAN_POINT ( 'NONE',  ( -2.625000000000000444, -28.29166666666666785, -4.546633369868303021 ) ) ;
#3650=ORIENTED_EDGE ( 'NONE', *, *, #4456, .F. ) ;
#3651=EDGE_LOOP ( 'NONE', ( #5998, #1417, #2871 ) ) ;
#3652=CARTESIAN_POINT ( 'NONE',  ( 5.250000000000000000, -29.62500000000000000, -6.429395695523604153E-16 ) ) ;
#3653=CARTESIAN_POINT ( 'NONE',  ( 5.385316468750000141, -27.23437499965860198, -6.595110575850215044E-16 ) ) ;
#3656=CARTESIAN_POINT ( 'NONE',  ( -1.406733260263389518, -27.98883544963257464, -5.250000000000001776 ) ) ;
#3659=CARTESIAN_POINT ( 'NONE',  ( 1.975475456537005874E-15, -27.37499999931720041, 5.250000000000000000 ) ) ;
#3667=CARTESIAN_POINT ( 'NONE',  ( -5.385316468749998364, -28.58854166632526983, 3.109213912904140287 ) ) ;
#3676=CARTESIAN_POINT ( 'NONE',  ( -5.250000000000000000, -29.50000000000000000, 0.000000000000000000 ) ) ;
#3678=CARTESIAN_POINT ( 'NONE',  ( -3.807688866302469071E-16, -27.64062499965859843, -6.218427825808274356 ) ) ;
#3692=ADVANCED_FACE ( 'NONE', ( #597 ), #7670, .F. ) ;
#3694=CARTESIAN_POINT ( 'NONE',  ( 2.625000000000002220, -27.16666666666666430, 4.546633369868302132 ) ) ;
#3698=ORIENTED_EDGE ( 'NONE', *, *, #7150, .T. ) ;
#3701=CARTESIAN_POINT ( 'NONE',  ( 5.385316468750000141, -27.48437499965860198, -6.595110575850215044E-16 ) ) ;
#3706=CARTESIAN_POINT ( 'NONE',  ( 1.975475456537005874E-15, -27.87499999931720041, 5.250000000000000000 ) ) ;
#3708=CARTESIAN_POINT ( 'NONE',  ( -2.692658234374996518, -27.56770833299193413, 4.663820869356208654 ) ) ;
#3712=CARTESIAN_POINT ( 'NONE',  ( 5.385316468750000141, -27.20312499965860198, -6.595110575850215044E-16 ) ) ;
#3715=CARTESIAN_POINT ( 'NONE',  ( 2.161402558328724325E-14, -29.49999999931720396, -5.250000000000000000 ) ) ;
#3718=CARTESIAN_POINT ( 'NONE',  ( -2.624999999999996891, -28.14583333265053255, 4.546633369868304797 ) ) ;
#3719=CARTESIAN_POINT ( 'NONE',  ( 2.624999999999998668, -27.58333333333333570, -4.546633369868303021 ) ) ;
#3721=VECTOR ( 'NONE', #2760, 1000.000000000000000 ) ;
#3722=CARTESIAN_POINT ( 'NONE',  ( 2.625000000000002220, -29.60416666598386826, 4.546633369868302132 ) ) ;
#3723=EDGE_CURVE ( 'NONE', #2779, #7570, #5575, .T. ) ;
#3724=ORIENTED_EDGE ( 'NONE', *, *, #1329, .T. ) ;
#3726=CARTESIAN_POINT ( 'NONE',  ( -3.807688866302469071E-16, -28.14062499965860198, -6.218427825808274356 ) ) ;
#3732=AXIS2_PLACEMENT_3D ( 'NONE', #9184, #7098, #722 ) ;
#3740=EDGE_CURVE ( 'NONE', #8455, #4014, #3087, .T. ) ;
#3744=CARTESIAN_POINT ( 'NONE',  ( 0.000000000000000000, -30.00000000000000000, -5.242490174541154069 ) ) ;
#3746=( NAMED_UNIT ( * ) PLANE_ANGLE_UNIT ( ) SI_UNIT ( $, .RADIAN. ) );
#3752=CARTESIAN_POINT ( 'NONE',  ( -5.385316468749998364, -27.83854166632526628, 3.109213912904140287 ) ) ;
#3756=CARTESIAN_POINT ( 'NONE',  ( 1.406733260263385521, -29.92633545031537068, 5.250000000000006217 ) ) ;
#3758=CARTESIAN_POINT ( 'NONE',  ( 5.385316468750001029, -27.75520833299194123, 3.109213912904135846 ) ) ;
#3761=CARTESIAN_POINT ( 'NONE',  ( -2.692658234375000514, -27.36979166632526628, -4.663820869356205989 ) ) ;
#3764=CARTESIAN_POINT ( 'NONE',  ( -1.406733260263391960, -27.38616454900182973, 5.250000000000000000 ) ) ;
#3768=CARTESIAN_POINT ( 'NONE',  ( 2.625000000000002220, -27.85416666598386826, 4.546633369868302132 ) ) ;
#3769=CARTESIAN_POINT ( 'NONE',  ( -5.249999999999999112, -27.70833333265053255, -3.031088913245534755 ) ) ;
#3773=CARTESIAN_POINT ( 'NONE',  ( -2.692658234374996518, -27.78645833299193413, 4.663820869356208654 ) ) ;
#3776=CARTESIAN_POINT ( 'NONE',  ( 2.161402558328724325E-14, -28.56250000000000000, -5.250000000000000000 ) ) ;
#3778=FACE_OUTER_BOUND ( 'NONE', #396, .T. ) ;
#3780=VERTEX_POINT ( 'NONE', #119 ) ;
#3782=VECTOR ( 'NONE', #2492, 1000.000000000000000 ) ;
#3789=CARTESIAN_POINT ( 'NONE',  ( -2.033577675846918216E-14, -29.87499999931720396, 5.250000000000000888 ) ) ;
#3792=DIRECTION ( 'NONE',  ( 0.000000000000000000, 0.000000000000000000, -1.000000000000000000 ) ) ;
#3798=EDGE_LOOP ( 'NONE', ( #8560, #7747 ) ) ;
#3799=CARTESIAN_POINT ( 'NONE',  ( -2.625000000000000444, -29.79166666666666785, -4.546633369868303021 ) ) ;
#3800=CARTESIAN_POINT ( 'NONE',  ( 2.692658234375002735, -27.52604166632526628, 4.663820869356205101 ) ) ;
#3804=CARTESIAN_POINT ( 'NONE',  ( 5.385316468749999252, -27.96354166632526628, -3.109213912904139399 ) ) ;
#3811=CARTESIAN_POINT ( 'NONE',  ( 1.113604000661152470E-15, -27.62499999931720396, 6.062177826491070398 ) ) ;
#3817=CARTESIAN_POINT ( 'NONE',  ( 1.142306659890740623E-15, -28.26562499965860198, 6.218427825808274356 ) ) ;
#3819=LINE ( 'NONE', #3260, #6360 ) ;
#3820=ORIENTED_EDGE ( 'NONE', *, *, #2854, .T. ) ;
#3821=CARTESIAN_POINT ( 'NONE',  ( 2.692658234374998738, -27.91145833299193413, -4.663820869356206877 ) ) ;
#3823=ORIENTED_EDGE ( 'NONE', *, *, #8661, .T. ) ;
#3827=CARTESIAN_POINT ( 'NONE',  ( -3.712013335537174572E-16, -27.31250000000000000, -6.062177826491070398 ) ) ;
#3834=ORIENTED_EDGE ( 'NONE', *, *, #1174, .T. ) ;
#3839=EDGE_CURVE ( 'NONE', #8840, #301, #1467, .T. ) ;
#3840=CARTESIAN_POINT ( 'NONE',  ( 2.161402558328724325E-14, -29.56250000000000355, -5.250000000000000000 ) ) ;
#3844=CARTESIAN_POINT ( 'NONE',  ( -5.385316468750000141, -28.35937499965860198, 0.000000000000000000 ) ) ;
#3849=CARTESIAN_POINT ( 'NONE',  ( -5.385316468750001029, -28.38020833299193058, -3.109213912904136734 ) ) ;
#3850=ADVANCED_FACE ( 'NONE', ( #2215 ), #9060, .T. ) ;
#3855=CARTESIAN_POINT ( 'NONE',  ( 2.161402558328724325E-14, -28.74999999931720751, -5.250000000000000000 ) ) ;
#3857=CYLINDRICAL_SURFACE ( 'NONE', #7714, 5.250000000000000000 ) ;
#3858=CARTESIAN_POINT ( 'NONE',  ( -2.625000000000000444, -28.22916666598386826, -4.546633369868303021 ) ) ;
#3864=CARTESIAN_POINT ( 'NONE',  ( -5.385316468750000141, -28.57812499965860198, 0.000000000000000000 ) ) ;
#3867=ORIENTED_EDGE ( 'NONE', *, *, #814, .F. ) ;
#3870=CARTESIAN_POINT ( 'NONE',  ( 5.385316468750000141, -27.95312499965860198, -6.595110575850215044E-16 ) ) ;
#3877=CARTESIAN_POINT ( 'NONE',  ( -2.625000000000000444, -27.54166666666666430, -4.546633369868303021 ) ) ;
#3885=( NAMED_UNIT ( * ) SI_UNIT ( $, .STERADIAN. ) SOLID_ANGLE_UNIT ( ) );
#3886=ADVANCED_FACE ( 'NONE', ( #3527 ), #166, .T. ) ;
#3891=CARTESIAN_POINT ( 'NONE',  ( 1.406733260263398400, -27.82366454968462932, -5.249999999999997335 ) ) ;
#3892=CARTESIAN_POINT ( 'NONE',  ( 5.385316468750000141, -28.73437499965860198, -6.595110575850215044E-16 ) ) ;
#3895=CARTESIAN_POINT ( 'NONE',  ( -5.385316468750001029, -29.63020833299193768, -3.109213912904136734 ) ) ;
#3899=CARTESIAN_POINT ( 'NONE',  ( -2.692658234374996518, -27.31770833299193413, 4.663820869356208654 ) ) ;
#3901=CARTESIAN_POINT ( 'NONE',  ( -2.692658234375000514, -27.86979166632526628, -4.663820869356205989 ) ) ;
#3905=CARTESIAN_POINT ( 'NONE',  ( 5.250000000000000000, -27.79166666598386826, -3.031088913245536531 ) ) ;
#3910=CARTESIAN_POINT ( 'NONE',  ( -3.807688866302469071E-16, -29.89062499965859843, -6.218427825808274356 ) ) ;
#3912=CARTESIAN_POINT ( 'NONE',  ( -1.406733260263384411, -28.55133545031537068, -5.250000000000006217 ) ) ;
#3915=CARTESIAN_POINT ( 'NONE',  ( -5.385316468750001029, -27.84895833299193413, -3.109213912904136734 ) ) ;
#3919=CARTESIAN_POINT ( 'NONE',  ( 5.250000000000000000, -27.12500000000000000, -6.429395695523604153E-16 ) ) ;
#3936=CARTESIAN_POINT ( 'NONE',  ( 5.385316468750001029, -29.25520833299193058, 3.109213912904134958 ) ) ;
#3937=CARTESIAN_POINT ( 'NONE',  ( -3.807688866302469071E-16, -29.92187499965859843, -6.218427825808274356 ) ) ;
#3939=CARTESIAN_POINT ( 'NONE',  ( -2.692658234374996518, -29.81770833299193413, 4.663820869356208654 ) ) ;
#3942=PRODUCT_DEFINITION ( 'UNKNOWN', '', #9030, #6845 ) ;
#3944=CARTESIAN_POINT ( 'NONE',  ( 2.692658234374998738, -29.69270833299193413, -4.663820869356206877 ) ) ;
#3947=CARTESIAN_POINT ( 'NONE',  ( 5.385316468749999252, -28.68229166632526983, -3.109213912904138954 ) ) ;
#3957=CARTESIAN_POINT ( 'NONE',  ( 5.385316468750001029, -29.97395833299194123, 3.109213912904135846 ) ) ;
#3960=CARTESIAN_POINT ( 'NONE',  ( 1.406733260263393293, -28.51116454900183328, -5.250000000000000000 ) ) ;
#3961=CARTESIAN_POINT ( 'NONE',  ( -2.692658234375000514, -28.61979166632526628, -4.663820869356205989 ) ) ;
#3963=VERTEX_POINT ( 'NONE', #98 ) ;
#3964=CARTESIAN_POINT ( 'NONE',  ( 1.113604000661152470E-15, -30.12499999931720041, 6.062177826491070398 ) ) ;
#3965=DIRECTION ( 'NONE',  ( 0.000000000000000000, -1.000000000000000000, 0.000000000000000000 ) ) ;
#3967=ORIENTED_EDGE ( 'NONE', *, *, #4861, .F. ) ;
#3968=FILL_AREA_STYLE_COLOUR ( '', #3094 ) ;
#3969=CARTESIAN_POINT ( 'NONE',  ( -3.712013335537174572E-16, -28.81249999999999645, -6.062177826491070398 ) ) ;
#3976=CARTESIAN_POINT ( 'NONE',  ( -2.033577675846918216E-14, -29.12499999931720751, 5.250000000000000888 ) ) ;
#3979=VERTEX_POINT ( 'NONE', #8008 ) ;
#3983=CARTESIAN_POINT ( 'NONE',  ( 5.385316468749999252, -29.46354166632526983, -3.109213912904138954 ) ) ;
#3985=DIRECTION ( 'NONE',  ( 0.000000000000000000, -1.000000000000000000, 0.000000000000000000 ) ) ;
#3987=CARTESIAN_POINT ( 'NONE',  ( 2.692658234375002735, -29.52604166632526983, 4.663820869356205101 ) ) ;
#3990=CARTESIAN_POINT ( 'NONE',  ( -5.249999999999999112, -27.52083333333333570, -3.031088913245534755 ) ) ;
#3992=CARTESIAN_POINT ( 'NONE',  ( 5.385316468749999252, -29.46354166632526983, -3.109213912904139399 ) ) ;
#3994=CARTESIAN_POINT ( 'NONE',  ( -3.807688866302469071E-16, -28.89062499965860198, -6.218427825808274356 ) ) ;
#3999=CARTESIAN_POINT ( 'NONE',  ( 5.250000000000000000, -27.37500000000000000, -6.429395695523604153E-16 ) ) ;
#4004=CARTESIAN_POINT ( 'NONE',  ( 5.385316468750000141, -29.70312499965859843, -6.595110575850215044E-16 ) ) ;
#4006=CARTESIAN_POINT ( 'NONE',  ( 2.625000000000002220, -28.60416666598386826, 4.546633369868302132 ) ) ;
#4007=CARTESIAN_POINT ( 'NONE',  ( 5.385316468750000141, -28.45312499965860198, -6.595110575850215044E-16 ) ) ;
#4010=CARTESIAN_POINT ( 'NONE',  ( 5.249999999999999112, -30.04166666598387181, -3.031088913245536975 ) ) ;
#4014=VERTEX_POINT ( 'NONE', #8705 ) ;
#4015=AXIS2_PLACEMENT_3D ( 'NONE', #6613, #241, #7360 ) ;
#4016=CARTESIAN_POINT ( 'NONE',  ( -5.249999999999999112, -28.47916666666666785, 3.031088913245538308 ) ) ;
#4026=CARTESIAN_POINT ( 'NONE',  ( 0.000000000000000000, 0.000000000000000000, 0.000000000000000000 ) ) ;
#4029=CARTESIAN_POINT ( 'NONE',  ( 5.250000000000000000, -27.87500000000000000, -6.429395695523604153E-16 ) ) ;
#4030=CARTESIAN_POINT ( 'NONE',  ( 2.692658234374998738, -28.69270833299193413, -4.663820869356206877 ) ) ;
#4033=CARTESIAN_POINT ( 'NONE',  ( 5.385316468749999252, -29.71354166632526983, -3.109213912904139399 ) ) ;
#4039=CARTESIAN_POINT ( 'NONE',  ( -1.406733260263391960, -27.44866454968463287, 5.250000000000000000 ) ) ;
#4041=CARTESIAN_POINT ( 'NONE',  ( 1.142306659890740623E-15, -29.79687499965859843, 6.218427825808274356 ) ) ;
#4043=CARTESIAN_POINT ( 'NONE',  ( 2.692658234374998738, -27.66145833299193413, -4.663820869356206877 ) ) ;
#4047=CARTESIAN_POINT ( 'NONE',  ( -5.249999999999997335, -28.41666666598386826, 3.031088913245538308 ) ) ;
#4049=CARTESIAN_POINT ( 'NONE',  ( 0.000000000000000000, -27.00000000000000000, -5.250000000000000000 ) ) ;
#4051=CARTESIAN_POINT ( 'NONE',  ( 5.385316468750000141, -29.45312499965859843, -6.595110575850215044E-16 ) ) ;
#4054=CARTESIAN_POINT ( 'NONE',  ( -5.385316468749998364, -29.30729166632526983, 3.109213912904140287 ) ) ;
#4061=CARTESIAN_POINT ( 'NONE',  ( -5.250000000000000000, -28.00000000000000000, 0.000000000000000000 ) ) ;
#4062=ORIENTED_EDGE ( 'NONE', *, *, #8843, .T. ) ;
#4065=DIRECTION ( 'NONE',  ( 0.000000000000000000, -1.000000000000000000, 0.000000000000000000 ) ) ;
#4073=CARTESIAN_POINT ( 'NONE',  ( -6.972266317189433020E-16, -29.81250000000000000, -5.249999999999999112 ) ) ;
#4074=CARTESIAN_POINT ( 'NONE',  ( 2.692658234375002735, -28.52604166632526628, 4.663820869356205101 ) ) ;
#4075=CARTESIAN_POINT ( 'NONE',  ( -5.385316468750000141, -29.85937499965859843, 0.000000000000000000 ) ) ;
#4078=CARTESIAN_POINT ( 'NONE',  ( 1.142306659890740623E-15, -29.04687499965859843, 6.218427825808274356 ) ) ;
#4085=CARTESIAN_POINT ( 'NONE',  ( 2.692658234375002735, -28.77604166632526628, 4.663820869356205101 ) ) ;
#4086=ORIENTED_EDGE ( 'NONE', *, *, #6301, .F. ) ;
#4087=CARTESIAN_POINT ( 'NONE',  ( -2.692658234375000514, -28.36979166632526628, -4.663820869356205989 ) ) ;
#4089=CARTESIAN_POINT ( 'NONE',  ( 0.000000000000000000, -30.00000000000000000, 0.000000000000000000 ) ) ;
#4096=CARTESIAN_POINT ( 'NONE',  ( -5.385316468750000141, -29.07812499965860198, 0.000000000000000000 ) ) ;
#4099=CARTESIAN_POINT ( 'NONE',  ( -1.406733260263391960, -29.44866454968462932, 5.250000000000000000 ) ) ;
#4100=CARTESIAN_POINT ( 'NONE',  ( 1.142306659890740623E-15, -27.29687499965859843, 6.218427825808274356 ) ) ;
#4106=CARTESIAN_POINT ( 'NONE',  ( 2.625000000000002220, -28.41666666666666785, 4.546633369868302132 ) ) ;
#4109=CARTESIAN_POINT ( 'NONE',  ( 2.624999999999998668, -28.08333333333333215, -4.546633369868303021 ) ) ;
#4114=CARTESIAN_POINT ( 'NONE',  ( 0.000000000000000000, -27.00000000000000000, 0.000000000000000000 ) ) ;
#4115=CARTESIAN_POINT ( 'NONE',  ( -5.249999999999999112, -28.66666666598386470, 3.031088913245538308 ) ) ;
#4116=CARTESIAN_POINT ( 'NONE',  ( -5.385316468750001029, -29.63020833299193768, -3.109213912904136734 ) ) ;
#4121=ORIENTED_EDGE ( 'NONE', *, *, #5300, .T. ) ;
#4122=CARTESIAN_POINT ( 'NONE',  ( -5.250000000000000000, -29.68749999931720041, 0.000000000000000000 ) ) ;
#4124=CARTESIAN_POINT ( 'NONE',  ( -5.385316468750000141, -28.60937499965860198, 0.000000000000000000 ) ) ;
#4125=EDGE_CURVE ( 'NONE', #1074, #2779, #4917, .T. ) ;
#4127=CARTESIAN_POINT ( 'NONE',  ( -5.385316468749998364, -29.05729166632526983, 3.109213912904140287 ) ) ;
#4133=ADVANCED_FACE ( 'NONE', ( #8558 ), #4422, .F. ) ;
#4136=CARTESIAN_POINT ( 'NONE',  ( 5.249999999999999112, -28.29166666598387181, -3.031088913245536975 ) ) ;
#4141=CARTESIAN_POINT ( 'NONE',  ( 0.000000000000000000, -27.00000000000000000, 0.000000000000000000 ) ) ;
#4142=CARTESIAN_POINT ( 'NONE',  ( -5.385316468750001029, -27.38020833299193768, -3.109213912904136734 ) ) ;
#4146=( BOUNDED_CURVE ( )  B_SPLINE_CURVE ( 2, ( #3855, #6678, #8777, #2267, #6633, #5889, #3113, #8728, #8683 ),
 .UNSPECIFIED., .F., .F. ) 
 B_SPLINE_CURVE_WITH_KNOTS ( ( 3, 2, 2, 2, 3 ),
 ( 0.5208333333333333703, 0.5277777777777777901, 0.5416666666666666297, 0.5555555555555555802, 0.5625000000000000000 ),
 .UNSPECIFIED. ) 
 CURVE ( )  GEOMETRIC_REPRESENTATION_ITEM ( )  RATIONAL_B_SPLINE_CURVE ( ( 0.9330127018922192983, 0.9330127018922198534, 1.000000000000000000, 0.8660254037844387076, 1.000000000000000000, 0.8660254037844387076, 1.000000000000000000, 0.9330127018922194093, 0.9330127018922194093 ) ) 
 REPRESENTATION_ITEM ( '' )  );
#4148=CARTESIAN_POINT ( 'NONE',  ( 5.250000000000000000, -28.85416666666666785, -3.031088913245536531 ) ) ;
#4160=DIRECTION ( 'NONE',  ( 0.000000000000000000, 0.000000000000000000, -1.000000000000000000 ) ) ;
#4162=CARTESIAN_POINT ( 'NONE',  ( 2.625000000000002220, -29.60416666598386826, 4.546633369868302132 ) ) ;
#4168=CARTESIAN_POINT ( 'NONE',  ( -6.972266317189433020E-16, -27.56249999999999645, -5.250000000000000000 ) ) ;
#4171=CARTESIAN_POINT ( 'NONE',  ( -2.625000000000000444, -27.22916666598386826, -4.546633369868303021 ) ) ;
#4173=CARTESIAN_POINT ( 'NONE',  ( 2.692658234375002735, -29.24479166632526983, 4.663820869356205101 ) ) ;
#4179=DIRECTION ( 'NONE',  ( -0.000000000000000000, 1.000000000000000000, -0.000000000000000000 ) ) ;
#4182=CARTESIAN_POINT ( 'NONE',  ( 2.625000000000002220, -28.35416666598386826, 4.546633369868302132 ) ) ;
#4186=CARTESIAN_POINT ( 'NONE',  ( 5.385316468750001029, -29.97395833299194123, 3.109213912904135846 ) ) ;
#4190=ADVANCED_FACE ( 'NONE', ( #3778 ), #7782, .T. ) ;
#4193=CARTESIAN_POINT ( 'NONE',  ( -2.692658234374996518, -27.28645833299193413, 4.663820869356208654 ) ) ;
#4199=( BOUNDED_CURVE ( )  B_SPLINE_CURVE ( 2, ( #9108, #4099, #1916, #1118, #1213, #2570, #6887, #8331, #5388 ),
 .UNSPECIFIED., .F., .F. ) 
 B_SPLINE_CURVE_WITH_KNOTS ( ( 3, 2, 2, 2, 3 ),
 ( 0.8125000000000000000, 0.8194444444444444198, 0.8333333333333333703, 0.8472222222222222099, 0.8541666666666667407 ),
 .UNSPECIFIED. ) 
 CURVE ( )  GEOMETRIC_REPRESENTATION_ITEM ( )  RATIONAL_B_SPLINE_CURVE ( ( 0.9330127018922194093, 0.9330127018922194093, 1.000000000000000000, 0.8660254037844387076, 1.000000000000000000, 0.8660254037844387076, 1.000000000000000000, 0.9330127018922187432, 0.9330127018922192983 ) ) 
 REPRESENTATION_ITEM ( '' )  );
#4204=CARTESIAN_POINT ( 'NONE',  ( 5.250000000000000888, -29.83333333265053966, 3.031088913245532979 ) ) ;
#4208=CARTESIAN_POINT ( 'NONE',  ( 6.429395695523604153E-16, -27.00000000000000000, 5.250000000000000000 ) ) ;
#4211=EDGE_CURVE ( 'NONE', #2331, #3224, #1368, .T. ) ;
#4218=CARTESIAN_POINT ( 'NONE',  ( -5.385316468750000141, -30.07812499965859843, 0.000000000000000000 ) ) ;
#4220=CARTESIAN_POINT ( 'NONE',  ( 0.000000000000000000, -27.00000000000000000, -5.250000000000000000 ) ) ;
#4222=AXIS2_PLACEMENT_3D ( 'NONE', #8897, #5411, #1185 ) ;
#4223=CARTESIAN_POINT ( 'NONE',  ( 6.429395695523604153E-16, -27.00000000000000000, 5.250000000000000000 ) ) ;
#4224=LINE ( 'NONE', #771, #5318 ) ;
#4229=CARTESIAN_POINT ( 'NONE',  ( 5.250000000000000888, -27.83333333265053611, 3.031088913245533423 ) ) ;
#4232=CARTESIAN_POINT ( 'NONE',  ( 1.142306659890740623E-15, -29.26562499965860198, 6.218427825808274356 ) ) ;
#4233=EDGE_CURVE ( 'NONE', #2823, #451, #5978, .T. ) ;
#4239=CARTESIAN_POINT ( 'NONE',  ( -3.712013335537174572E-16, -29.31249999999999645, -6.062177826491070398 ) ) ;
#4243=FACE_BOUND ( 'NONE', #1146, .T. ) ;
#4247=CARTESIAN_POINT ( 'NONE',  ( 5.250000000000000888, -29.08333333265053611, 3.031088913245532979 ) ) ;
#4248=( BOUNDED_CURVE ( )  B_SPLINE_CURVE ( 2, ( #6207, #8396, #1407, #577, #663, #9166, #6910, #5636, #6949 ),
 .UNSPECIFIED., .F., .F. ) 
 B_SPLINE_CURVE_WITH_KNOTS ( ( 3, 2, 2, 2, 3 ),
 ( 0.7291666666666667407, 0.7361111111111111605, 0.7500000000000000000, 0.7638888888888888395, 0.7708333333333333703 ),
 .UNSPECIFIED. ) 
 CURVE ( )  GEOMETRIC_REPRESENTATION_ITEM ( )  RATIONAL_B_SPLINE_CURVE ( ( 0.9330127018922192983, 0.9330127018922198534, 1.000000000000000000, 0.8660254037844387076, 1.000000000000000000, 0.8660254037844387076, 1.000000000000000000, 0.9330127018922187432, 0.9330127018922192983 ) ) 
 REPRESENTATION_ITEM ( '' )  );
#4257=ORIENTED_EDGE ( 'NONE', *, *, #3723, .T. ) ;
#4258=CARTESIAN_POINT ( 'NONE',  ( -2.692658234374996518, -29.03645833299193413, 4.663820869356208654 ) ) ;
#4260=LINE ( 'NONE', #767, #8895 ) ;
#4263=CARTESIAN_POINT ( 'NONE',  ( 0.000000000000000000, -50.00000000000000000, 0.000000000000000000 ) ) ;
#4265=CARTESIAN_POINT ( 'NONE',  ( 5.250000000000000000, -28.87499999999999645, -6.429395695523604153E-16 ) ) ;
#4267=DIRECTION ( 'NONE',  ( 0.000000000000000000, -1.000000000000000000, 0.000000000000000000 ) ) ;
#4272=STYLED_ITEM ( 'NONE', ( #6150 ), #3635 ) ;
#4274=CARTESIAN_POINT ( 'NONE',  ( 2.692658234374998738, -27.44270833299193413, -4.663820869356206877 ) ) ;
#4282=CARTESIAN_POINT ( 'NONE',  ( 2.625000000000002220, -29.16666666666666785, 4.546633369868302132 ) ) ;
#4283=DIRECTION ( 'NONE',  ( 0.000000000000000000, 0.000000000000000000, -1.000000000000000000 ) ) ;
#4285=EDGE_LOOP ( 'NONE', ( #4086, #5177, #8194, #86 ) ) ;
#4287=DIRECTION ( 'NONE',  ( -0.000000000000000000, 1.000000000000000000, -0.000000000000000000 ) ) ;
#4291=CARTESIAN_POINT ( 'NONE',  ( -5.250000000000000000, -29.68749999931720041, 0.000000000000000000 ) ) ;
#4294=DIRECTION ( 'NONE',  ( 0.000000000000000000, 0.000000000000000000, -1.000000000000000000 ) ) ;
#4300=CARTESIAN_POINT ( 'NONE',  ( -1.406733260263384411, -29.73883544963257108, -5.250000000000006217 ) ) ;
#4305=AXIS2_PLACEMENT_3D ( 'NONE', #8307, #4677, #1098 ) ;
#4306=CARTESIAN_POINT ( 'NONE',  ( -5.385316468750001029, -29.84895833299193413, -3.109213912904136734 ) ) ;
#4311=CARTESIAN_POINT ( 'NONE',  ( -2.033577675846918216E-14, -28.93750000000000000, 5.250000000000000888 ) ) ;
#4313=CARTESIAN_POINT ( 'NONE',  ( 5.385316468749999252, -27.21354166632526628, -3.109213912904139399 ) ) ;
#4319=CARTESIAN_POINT ( 'NONE',  ( 1.142306659890740623E-15, -27.79687499965860198, 6.218427825808274356 ) ) ;
#4327=CARTESIAN_POINT ( 'NONE',  ( -5.385316468750000141, -27.32812499965860198, 0.000000000000000000 ) ) ;
#4328=ORIENTED_EDGE ( 'NONE', *, *, #5626, .T. ) ;
#4332=ORIENTED_EDGE ( 'NONE', *, *, #5112, .T. ) ;
#4337=CARTESIAN_POINT ( 'NONE',  ( -5.250000000000000000, -29.93749999931720041, 0.000000000000000000 ) ) ;
#4340=CARTESIAN_POINT ( 'NONE',  ( 1.975475456537005874E-15, -27.68749999999999289, 5.250000000000000000 ) ) ;
#4343=ADVANCED_FACE ( 'NONE', ( #1279 ), #2775, .T. ) ;
#4351=EDGE_CURVE ( 'NONE', #301, #7570, #60, .T. ) ;
#4352=CARTESIAN_POINT ( 'NONE',  ( -5.249999999999997335, -29.72916666666666430, 3.031088913245538308 ) ) ;
#4353=CARTESIAN_POINT ( 'NONE',  ( 5.385316468749999252, -27.46354166632526628, -3.109213912904138954 ) ) ;
#4355=VECTOR ( 'NONE', #6243, 1000.000000000000000 ) ;
#4364=CARTESIAN_POINT ( 'NONE',  ( -3.807688866302469071E-16, -27.14062499965860198, -6.218427825808274356 ) ) ;
#4366=CARTESIAN_POINT ( 'NONE',  ( -3.807688866302469071E-16, -27.67187499965859843, -6.218427825808274356 ) ) ;
#4372=CYLINDRICAL_SURFACE ( 'NONE', #4455, 5.250000000000000000 ) ;
#4374=CARTESIAN_POINT ( 'NONE',  ( -5.250000000000000000, -29.27083333333333215, -3.031088913245534755 ) ) ;
#4376=CARTESIAN_POINT ( 'NONE',  ( 2.692658234375002735, -27.49479166632526628, 4.663820869356205101 ) ) ;
#4391=EDGE_LOOP ( 'NONE', ( #3317, #2284, #6338, #3514 ) ) ;
#4392=CARTESIAN_POINT ( 'NONE',  ( 2.624999999999998668, -27.08333333333333570, -4.546633369868303021 ) ) ;
#4395=VERTEX_POINT ( 'NONE', #2728 ) ;
#4401=EDGE_CURVE ( 'NONE', #7820, #8840, #6179, .T. ) ;
#4404=CARTESIAN_POINT ( 'NONE',  ( -2.692658234374996518, -28.56770833299193413, 4.663820869356208654 ) ) ;
#4405=UNCERTAINTY_MEASURE_WITH_UNIT (LENGTH_MEASURE( 1.000000000000000082E-05 ), #6796, 'distance_accuracy_value', 'NONE');
#4410=CARTESIAN_POINT ( 'NONE',  ( -2.625000000000000444, -29.47916666598386826, -4.546633369868303021 ) ) ;
#4413=CARTESIAN_POINT ( 'NONE',  ( 2.625000000000002220, -28.10416666598386826, 4.546633369868302132 ) ) ;
#4414=CARTESIAN_POINT ( 'NONE',  ( -2.625000000000000444, -27.72916666598386826, -4.546633369868303021 ) ) ;
#4417=CARTESIAN_POINT ( 'NONE',  ( 2.625000000000002220, -29.85416666598387181, 4.546633369868302132 ) ) ;
#4418=EDGE_LOOP ( 'NONE', ( #7417, #3410, #1679, #6191 ) ) ;
#4419=CARTESIAN_POINT ( 'NONE',  ( -5.385316468750001029, -27.59895833299193413, -3.109213912904136734 ) ) ;
#4422=CYLINDRICAL_SURFACE ( 'NONE', #5382, 5.250000000000000000 ) ;
#4424=EDGE_LOOP ( 'NONE', ( #1463, #3632, #7619, #5278 ) ) ;
#4427=CARTESIAN_POINT ( 'NONE',  ( 5.250000000000000000, -27.12500000000000000, -6.429395695523604153E-16 ) ) ;
#4428=CARTESIAN_POINT ( 'NONE',  ( -2.625000000000000444, -29.97916666598387181, -4.546633369868303021 ) ) ;
#4434=ORIENTED_EDGE ( 'NONE', *, *, #2572, .F. ) ;
#4438=AXIS2_PLACEMENT_3D ( 'NONE', #3216, #6737, #4465 ) ;
#4441=CARTESIAN_POINT ( 'NONE',  ( 1.142306659890740623E-15, -27.54687499965860198, 6.218427825808274356 ) ) ;
#4443=DIRECTION ( 'NONE',  ( -0.000000000000000000, 1.000000000000000000, -0.000000000000000000 ) ) ;
#4444=ORIENTED_EDGE ( 'NONE', *, *, #8843, .F. ) ;
#4445=CARTESIAN_POINT ( 'NONE',  ( 1.975475456537005874E-15, -27.93749999999999289, 5.249999999999999112 ) ) ;
#4447=CARTESIAN_POINT ( 'NONE',  ( -2.692658234374996518, -28.06770833299193413, 4.663820869356208654 ) ) ;
#4450=CARTESIAN_POINT ( 'NONE',  ( 2.692658234375002735, -27.49479166632526628, 4.663820869356205101 ) ) ;
#4453=DIRECTION ( 'NONE',  ( 0.000000000000000000, -1.000000000000000000, 0.000000000000000000 ) ) ;
#4455=AXIS2_PLACEMENT_3D ( 'NONE', #314, #8089, #5150 ) ;
#4456=EDGE_CURVE ( 'NONE', #4617, #2202, #7121, .T. ) ;
#4457=CARTESIAN_POINT ( 'NONE',  ( 5.250000000000000000, -27.31249999931720396, -6.429395695523604153E-16 ) ) ;
#4461=CARTESIAN_POINT ( 'NONE',  ( 2.161402558328724325E-14, -29.74999999931720396, -5.250000000000000000 ) ) ;
#4463=CARTESIAN_POINT ( 'NONE',  ( -5.385316468750000141, -28.32812499965860198, 0.000000000000000000 ) ) ;
#4465=DIRECTION ( 'NONE',  ( 0.000000000000000000, 0.000000000000000000, -1.000000000000000000 ) ) ;
#4467=CARTESIAN_POINT ( 'NONE',  ( 2.692658234374998738, -27.16145833299193413, -4.663820869356206877 ) ) ;
#4469=ORIENTED_EDGE ( 'NONE', *, *, #8173, .F. ) ;
#4480=CARTESIAN_POINT ( 'NONE',  ( -1.406733220335620871, -29.98883544994945538, -5.250000023052310283 ) ) ;
#4485=EDGE_CURVE ( 'NONE', #3224, #1598, #5915, .T. ) ;
#4486=CARTESIAN_POINT ( 'NONE',  ( 1.975475456537005874E-15, -28.12499999931720041, 5.250000000000000000 ) ) ;
#4489=EDGE_CURVE ( 'NONE', #3220, #946, #7342, .T. ) ;
#4491=DIRECTION ( 'NONE',  ( 0.000000000000000000, -1.000000000000000000, 0.000000000000000000 ) ) ;
#4492=CARTESIAN_POINT ( 'NONE',  ( 5.385316468749999252, -27.71354166632526272, -3.109213912904138954 ) ) ;
#4496=VERTEX_POINT ( 'NONE', #5823 ) ;
#4498=CARTESIAN_POINT ( 'NONE',  ( -2.033577675846918216E-14, -29.93750000000000355, 5.250000000000000888 ) ) ;
#4500=CARTESIAN_POINT ( 'NONE',  ( -5.385316468749998364, -27.83854166632526628, 3.109213912904140287 ) ) ;
#4503=VERTEX_POINT ( 'NONE', #3744 ) ;
#4504=CARTESIAN_POINT ( 'NONE',  ( -5.385316468750001029, -27.59895833299194123, -3.109213912904136734 ) ) ;
#4509=VECTOR ( 'NONE', #5770, 1000.000000000000114 ) ;
#4510=CARTESIAN_POINT ( 'NONE',  ( -2.624999999999996891, -27.64583333265053611, 4.546633369868304797 ) ) ;
#4511=CARTESIAN_POINT ( 'NONE',  ( -6.972266317189433020E-16, -27.06250000000000000, -5.250000000000000000 ) ) ;
#4515=CARTESIAN_POINT ( 'NONE',  ( 5.385316468750001029, -27.72395833299193413, 3.109213912904135846 ) ) ;
#4520=CARTESIAN_POINT ( 'NONE',  ( -5.385316468750001029, -28.84895833299193413, -3.109213912904136734 ) ) ;
#4522=EDGE_LOOP ( 'NONE', ( #1355, #7638, #523, #8955 ) ) ;
#4524=EDGE_CURVE ( 'NONE', #4744, #7091, #4930, .T. ) ;
#4526=CARTESIAN_POINT ( 'NONE',  ( 5.250000000000000000, -27.62500000000000000, -6.429395695523604153E-16 ) ) ;
#4527=CARTESIAN_POINT ( 'NONE',  ( 5.250000000000000888, -30.08333333265053255, 3.031088913245532979 ) ) ;
#4537=CARTESIAN_POINT ( 'NONE',  ( -5.385316468749998364, -27.58854166632526628, 3.109213912904140287 ) ) ;
#4540=CARTESIAN_POINT ( 'NONE',  ( -6.972266317189433020E-16, -29.24999999931720396, -5.250000000000000000 ) ) ;
#4541=CARTESIAN_POINT ( 'NONE',  ( -5.385316468750001029, -28.13020833299193058, -3.109213912904136734 ) ) ;
#4543=CARTESIAN_POINT ( 'NONE',  ( 2.625000000000002220, -29.91666666666666785, 4.546633369868302132 ) ) ;
#4545=CARTESIAN_POINT ( 'NONE',  ( 5.385316468749999252, -27.46354166632526983, -3.109213912904139399 ) ) ;
#4550=FACE_OUTER_BOUND ( 'NONE', #5562, .T. ) ;
#4552=CARTESIAN_POINT ( 'NONE',  ( 5.250000000000000888, -27.83333333265053611, 3.031088913245532979 ) ) ;
#4555=CARTESIAN_POINT ( 'NONE',  ( -2.033577675846918216E-14, -29.18750000000000000, 5.250000000000000888 ) ) ;
#4556=ORIENTED_EDGE ( 'NONE', *, *, #6707, .F. ) ;
#4557=CARTESIAN_POINT ( 'NONE',  ( 2.692658234375002735, -28.49479166632526628, 4.663820869356205101 ) ) ;
#4562=CARTESIAN_POINT ( 'NONE',  ( -5.385316468750000141, -28.32812499965860198, 0.000000000000000000 ) ) ;
#4573=CARTESIAN_POINT ( 'NONE',  ( 1.406733260263403507, -29.51116454900182973, -5.249999999999994671 ) ) ;
#4577=FACE_OUTER_BOUND ( 'NONE', #757, .T. ) ;
#4583=CARTESIAN_POINT ( 'NONE',  ( -3.807688866302469071E-16, -28.92187499965859487, -6.218427825808274356 ) ) ;
#4586=CARTESIAN_POINT ( 'NONE',  ( -5.385316468749998364, -28.08854166632526628, 3.109213912904140287 ) ) ;
#4587=ORIENTED_EDGE ( 'NONE', *, *, #6878, .F. ) ;
#4591=CARTESIAN_POINT ( 'NONE',  ( -2.692658234375000514, -27.40104166632526628, -4.663820869356205989 ) ) ;
#4593=CONICAL_SURFACE ( 'NONE', #586, 5.257453848358681014, 0.1221730476396033355 ) ;
#4594=CARTESIAN_POINT ( 'NONE',  ( -5.385316468750001029, -28.34895833299193413, -3.109213912904136734 ) ) ;
#4596=CARTESIAN_POINT ( 'NONE',  ( 2.324088772396477476E-15, -27.49999999931720751, -5.250000000000000000 ) ) ;
#4598=CARTESIAN_POINT ( 'NONE',  ( 5.250000000000000888, -28.33333333265053611, 3.031088913245532979 ) ) ;
#4599=CARTESIAN_POINT ( 'NONE',  ( -2.624999999999996891, -27.64583333265053611, 4.546633369868304797 ) ) ;
#4602=ORIENTED_EDGE ( 'NONE', *, *, #5006, .T. ) ;
#4604=CARTESIAN_POINT ( 'NONE',  ( 5.385316468750001029, -27.97395833299193413, 3.109213912904135846 ) ) ;
#4609=CARTESIAN_POINT ( 'NONE',  ( -5.385316468750001029, -28.09895833299193413, -3.109213912904136734 ) ) ;
#4617=VERTEX_POINT ( 'NONE', #5451 ) ;
#4620=CARTESIAN_POINT ( 'NONE',  ( 6.972266317189434006E-16, -27.24999999931720751, -5.250000000000000000 ) ) ;
#4626=( BOUNDED_CURVE ( )  B_SPLINE_CURVE ( 2, ( #2115, #6428, #2825, #20, #5688, #8533, #4940, #9091, #64 ),
 .UNSPECIFIED., .F., .F. ) 
 B_SPLINE_CURVE_WITH_KNOTS ( ( 3, 2, 2, 2, 3 ),
 ( 0.5625000000000000000, 0.5694444444444444198, 0.5833333333333333703, 0.5972222222222222099, 0.6041666666666667407 ),
 .UNSPECIFIED. ) 
 CURVE ( )  GEOMETRIC_REPRESENTATION_ITEM ( )  RATIONAL_B_SPLINE_CURVE ( ( 0.9330127018922194093, 0.9330127018922194093, 1.000000000000000000, 0.8660254037844387076, 1.000000000000000000, 0.8660254037844387076, 1.000000000000000000, 0.9330127018922187432, 0.9330127018922192983 ) ) 
 REPRESENTATION_ITEM ( '' )  );
#4629=CARTESIAN_POINT ( 'NONE',  ( 5.385316468750001029, -28.50520833299193058, 3.109213912904134958 ) ) ;
#4632=CARTESIAN_POINT ( 'NONE',  ( -2.692658234375000514, -29.40104166632526983, -4.663820869356205989 ) ) ;
#4633=ORIENTED_EDGE ( 'NONE', *, *, #3740, .F. ) ;
#4634=CARTESIAN_POINT ( 'NONE',  ( -6.972266317189433020E-16, -28.31249999999999645, -5.250000000000000000 ) ) ;
#4636=CARTESIAN_POINT ( 'NONE',  ( 2.692658234375002735, -29.27604166632526983, 4.663820869356205101 ) ) ;
#4639=CARTESIAN_POINT ( 'NONE',  ( 5.385316468749999252, -27.68229166632526272, -3.109213912904138954 ) ) ;
#4648=PRODUCT_CONTEXT ( 'NONE', #8005, 'mechanical' ) ;
#4649=CARTESIAN_POINT ( 'NONE',  ( -5.385316468750001029, -29.84895833299193413, -3.109213912904136734 ) ) ;
#4651=CARTESIAN_POINT ( 'NONE',  ( 5.385316468750001029, -27.72395833299193413, 3.109213912904135846 ) ) ;
#4659=ADVANCED_FACE ( 'NONE', ( #3369 ), #3275, .F. ) ;
#4662=CARTESIAN_POINT ( 'NONE',  ( 5.250000000000000000, -28.62500000000000000, -6.429395695523604153E-16 ) ) ;
#4675=CARTESIAN_POINT ( 'NONE',  ( 5.385316468750001029, -29.00520833299193413, 3.109213912904134958 ) ) ;
#4677=DIRECTION ( 'NONE',  ( 0.000000000000000000, -1.000000000000000000, 0.000000000000000000 ) ) ;
#4678=CARTESIAN_POINT ( 'NONE',  ( -3.807688866302469071E-16, -28.92187499965860198, -6.218427825808274356 ) ) ;
#4683=CARTESIAN_POINT ( 'NONE',  ( 1.142306659890740623E-15, -29.04687499965859843, 6.218427825808274356 ) ) ;
#4684=ORIENTED_EDGE ( 'NONE', *, *, #2568, .F. ) ;
#4685=CARTESIAN_POINT ( 'NONE',  ( 2.692658234374998738, -28.16145833299193413, -4.663820869356206877 ) ) ;
#4694=CARTESIAN_POINT ( 'NONE',  ( 5.385316468750000141, -28.95312499965860198, -6.595110575850215044E-16 ) ) ;
#4697=CARTESIAN_POINT ( 'NONE',  ( -5.385316468750000141, -28.82812499965860198, 0.000000000000000000 ) ) ;
#4703=EDGE_CURVE ( 'NONE', #8050, #4395, #8219, .T. ) ;
#4705=ORIENTED_EDGE ( 'NONE', *, *, #4754, .F. ) ;
#4707=CARTESIAN_POINT ( 'NONE',  ( -3.712013335537174572E-16, -29.06250000000000000, -6.062177826491070398 ) ) ;
#4708=ORIENTED_EDGE ( 'NONE', *, *, #8041, .F. ) ;
#4711=DIRECTION ( 'NONE',  ( 0.000000000000000000, -1.000000000000000000, 0.000000000000000000 ) ) ;
#4719=CARTESIAN_POINT ( 'NONE',  ( 5.385316468749999252, -28.46354166632526628, -3.109213912904138954 ) ) ;
#4722=CARTESIAN_POINT ( 'NONE',  ( 5.385316468749999252, -29.46354166632526983, -3.109213912904139399 ) ) ;
#4728=CARTESIAN_POINT ( 'NONE',  ( 5.385316468749999252, -29.71354166632526983, -3.109213912904139399 ) ) ;
#4730=CARTESIAN_POINT ( 'NONE',  ( 1.142306659890740623E-15, -28.01562499965859843, 6.218427825808274356 ) ) ;
#4732=CARTESIAN_POINT ( 'NONE',  ( -6.972266317189433020E-16, -28.31249999999999645, -5.249999999999999112 ) ) ;
#4738=CARTESIAN_POINT ( 'NONE',  ( 5.385316468750001029, -29.47395833299193413, 3.109213912904135846 ) ) ;
#4740=CARTESIAN_POINT ( 'NONE',  ( 1.406733260263390628, -28.61383544963257108, 5.250000000000001776 ) ) ;
#4741=CARTESIAN_POINT ( 'NONE',  ( -5.385316468749998364, -29.05729166632526628, 3.109213912904140287 ) ) ;
#4744=VERTEX_POINT ( 'NONE', #8159 ) ;
#4752=CARTESIAN_POINT ( 'NONE',  ( -2.624999999999996891, -28.70833333333333215, 4.546633369868304797 ) ) ;
#4754=EDGE_CURVE ( 'NONE', #8128, #946, #427, .T. ) ;
#4765=CARTESIAN_POINT ( 'NONE',  ( 5.385316468749999252, -28.71354166632526272, -3.109213912904138954 ) ) ;
#4766=FACE_OUTER_BOUND ( 'NONE', #8557, .T. ) ;
#4768=CARTESIAN_POINT ( 'NONE',  ( -2.692658234374996518, -29.06770833299193413, 4.663820869356208654 ) ) ;
#4772=CARTESIAN_POINT ( 'NONE',  ( 1.406733260263393293, -28.32366454968462932, -5.250000000000000000 ) ) ;
#4774=EDGE_CURVE ( 'NONE', #8385, #8796, #6941, .T. ) ;
#4775=CARTESIAN_POINT ( 'NONE',  ( -3.807688866302469071E-16, -28.92187499965860198, -6.218427825808274356 ) ) ;
#4778=CARTESIAN_POINT ( 'NONE',  ( -2.692658234375000514, -28.11979166632526628, -4.663820869356205989 ) ) ;
#4786=CARTESIAN_POINT ( 'NONE',  ( -5.385316468750001029, -29.09895833299193058, -3.109213912904136734 ) ) ;
#4789=CARTESIAN_POINT ( 'NONE',  ( -2.692658234375000514, -27.15104166632526628, -4.663820869356205989 ) ) ;
#4794=EDGE_LOOP ( 'NONE', ( #2401, #4469, #291, #4328 ) ) ;
#4795=( NAMED_UNIT ( * ) SI_UNIT ( $, .STERADIAN. ) SOLID_ANGLE_UNIT ( ) );
#4796=CARTESIAN_POINT ( 'NONE',  ( 2.625000000000002220, -28.66666666666666785, 4.546633369868302132 ) ) ;
#4803=EDGE_CURVE ( 'NONE', #4496, #4617, #7401, .T. ) ;
#4807=CARTESIAN_POINT ( 'NONE',  ( -1.406733260263384411, -28.80133545031537068, -5.250000000000006217 ) ) ;
#4808=CARTESIAN_POINT ( 'NONE',  ( -2.624999999999996891, -28.89583333265053611, 4.546633369868304797 ) ) ;
#4812=CARTESIAN_POINT ( 'NONE',  ( -2.692658234375000514, -29.90104166632526983, -4.663820869356205989 ) ) ;
#4819=CARTESIAN_POINT ( 'NONE',  ( 1.142306659890740623E-15, -28.79687499965860198, 6.218427825808274356 ) ) ;
#4821=CARTESIAN_POINT ( 'NONE',  ( -3.807688866302469071E-16, -29.14062499965860553, -6.218427825808274356 ) ) ;
#4827=CARTESIAN_POINT ( 'NONE',  ( 5.250000000000000000, -28.31249999931720396, -6.429395695523604153E-16 ) ) ;
#4829=CARTESIAN_POINT ( 'NONE',  ( -5.385316468750000141, -29.57812499965859843, 0.000000000000000000 ) ) ;
#4831=CARTESIAN_POINT ( 'NONE',  ( -2.624999999999996891, -27.95833333333333215, 4.546633369868304797 ) ) ;
#4832=CARTESIAN_POINT ( 'NONE',  ( 5.385316468749999252, -29.18229166632526983, -3.109213912904139399 ) ) ;
#4837=ORIENTED_EDGE ( 'NONE', *, *, #1228, .F. ) ;
#4838=CARTESIAN_POINT ( 'NONE',  ( -2.625000000000000444, -28.29166666666666785, -4.546633369868303021 ) ) ;
#4842=CYLINDRICAL_SURFACE ( 'NONE', #190, 5.250000000000000000 ) ;
#4847=LINE ( 'NONE', #7955, #279 ) ;
#4848=CARTESIAN_POINT ( 'NONE',  ( 2.624999999999998668, -29.02083333265053611, -4.546633369868303021 ) ) ;
#4850=CARTESIAN_POINT ( 'NONE',  ( -5.250000000000000000, -27.18749999931720396, 0.000000000000000000 ) ) ;
#4853=ORIENTED_EDGE ( 'NONE', *, *, #3049, .F. ) ;
#4856=CARTESIAN_POINT ( 'NONE',  ( 5.385316468750001029, -30.00520833299193768, 3.109213912904135846 ) ) ;
#4857=VERTEX_POINT ( 'NONE', #160 ) ;
#4858=CARTESIAN_POINT ( 'NONE',  ( 2.692658234374998738, -29.91145833299193413, -4.663820869356206877 ) ) ;
#4860=LINE ( 'NONE', #4220, #5488 ) ;
#4861=EDGE_CURVE ( 'NONE', #6553, #6037, #6437, .T. ) ;
#4868=CARTESIAN_POINT ( 'NONE',  ( 2.692658234374998738, -28.44270833299193413, -4.663820869356206877 ) ) ;
#4871=EDGE_CURVE ( 'NONE', #3470, #3226, #1979, .T. ) ;
#4873=CARTESIAN_POINT ( 'NONE',  ( -5.385316468750001029, -29.84895833299193413, -3.109213912904136734 ) ) ;
#4880=CARTESIAN_POINT ( 'NONE',  ( 5.385316468750000141, -27.20312499965860198, -6.595110575850215044E-16 ) ) ;
#4884=DIRECTION ( 'NONE',  ( 0.000000000000000000, -1.000000000000000000, 0.000000000000000000 ) ) ;
#4891=CARTESIAN_POINT ( 'NONE',  ( 2.624999999999998668, -29.52083333265053611, -4.546633369868303021 ) ) ;
#4896=ORIENTED_EDGE ( 'NONE', *, *, #7076, .F. ) ;
#4902=CARTESIAN_POINT ( 'NONE',  ( 5.385316468750000141, -29.45312499965859843, -6.595110575850215044E-16 ) ) ;
#4908=CARTESIAN_POINT ( 'NONE',  ( -5.250000000000000000, -27.09374999965859843, 0.000000000000000000 ) ) ;
#4913=CARTESIAN_POINT ( 'NONE',  ( 1.045839947578414884E-14, -28.24999999931720041, -5.250000000000000000 ) ) ;
#4914=CARTESIAN_POINT ( 'NONE',  ( 2.161402558328724325E-14, -28.74999999931720751, -5.250000000000000000 ) ) ;
#4916=CARTESIAN_POINT ( 'NONE',  ( 2.624999999999998668, -28.58333333333333215, -4.546633369868303021 ) ) ;
#4917=( BOUNDED_CURVE ( )  B_SPLINE_CURVE ( 2, ( #7162, #7864, #928, #3082, #5157, #1533, #2282, #739, #1485 ),
 .UNSPECIFIED., .F., .F. ) 
 B_SPLINE_CURVE_WITH_KNOTS ( ( 3, 2, 2, 2, 3 ),
 ( 0.06250000000000000000, 0.06944444444444444753, 0.08333333333333332871, 0.09722222222222222376, 0.1041666666666666713 ),
 .UNSPECIFIED. ) 
 CURVE ( )  GEOMETRIC_REPRESENTATION_ITEM ( )  RATIONAL_B_SPLINE_CURVE ( ( 0.9330127018922194093, 0.9330127018922194093, 1.000000000000000000, 0.8660254037844387076, 1.000000000000000000, 0.8660254037844387076, 1.000000000000000000, 0.9330127018922192983, 0.9330127018922194093 ) ) 
 REPRESENTATION_ITEM ( '' )  );
#4918=CARTESIAN_POINT ( 'NONE',  ( 1.142306659890740623E-15, -29.51562499965859487, 6.218427825808274356 ) ) ;
#4923=CARTESIAN_POINT ( 'NONE',  ( -5.249999999999999112, -29.47916666666666785, 3.031088913245538308 ) ) ;
#4930=CIRCLE ( 'NONE', #2271, 3.794308781941904574 ) ;
#4933=CARTESIAN_POINT ( 'NONE',  ( -5.249999999999999112, -28.91666666598386826, 3.031088913245538308 ) ) ;
#4936=DIRECTION ( 'NONE',  ( 0.000000000000000000, -1.000000000000000000, 0.000000000000000000 ) ) ;
#4940=CARTESIAN_POINT ( 'NONE',  ( -2.625000000000000444, -28.97916666598386826, -4.546633369868303021 ) ) ;
#4944=ORIENTED_EDGE ( 'NONE', *, *, #2626, .T. ) ;
#4945=CARTESIAN_POINT ( 'NONE',  ( -5.385316468749998364, -30.05729166632526628, 3.109213912904140287 ) ) ;
#4951=CARTESIAN_POINT ( 'NONE',  ( 5.385316468750000141, -27.23437499965860198, -6.595110575850215044E-16 ) ) ;
#4953=DIRECTION ( 'NONE',  ( 0.000000000000000000, 0.000000000000000000, -1.000000000000000000 ) ) ;
#4957=ADVANCED_FACE ( 'NONE', ( #4766 ), #3509, .F. ) ;
#4958=CARTESIAN_POINT ( 'NONE',  ( 1.142306659890740623E-15, -28.54687499965860198, 6.218427825808274356 ) ) ;
#4960=DIRECTION ( 'NONE',  ( 0.000000000000000000, -1.000000000000000000, 0.000000000000000000 ) ) ;
#4965=CARTESIAN_POINT ( 'NONE',  ( 2.624999999999998668, -29.33333333333333215, -4.546633369868303021 ) ) ;
#4966=EDGE_CURVE ( 'NONE', #8840, #2779, #6332, .T. ) ;
#4969=ORIENTED_EDGE ( 'NONE', *, *, #4803, .F. ) ;
#4974=CARTESIAN_POINT ( 'NONE',  ( 1.113604000661152470E-15, -29.87499999931720396, 6.062177826491070398 ) ) ;
#4985=CARTESIAN_POINT ( 'NONE',  ( -5.385316468749998364, -29.30729166632526983, 3.109213912904140287 ) ) ;
#4989=PRODUCT_DEFINITION_SHAPE ( 'NONE', 'NONE',  #3942 ) ;
#4990=CARTESIAN_POINT ( 'NONE',  ( -1.406733260263402174, -28.94866454968462577, 5.249999999999995559 ) ) ;
#4997=CARTESIAN_POINT ( 'NONE',  ( 2.161402558328724325E-14, -29.74999999931720396, -5.250000000000000000 ) ) ;
#4999=CARTESIAN_POINT ( 'NONE',  ( -5.385316468750000141, -27.60937499965860198, 0.000000000000000000 ) ) ;
#5001=DIRECTION ( 'NONE',  ( 0.000000000000000000, 0.000000000000000000, -1.000000000000000000 ) ) ;
#5003=ORIENTED_EDGE ( 'NONE', *, *, #7886, .T. ) ;
#5005=CARTESIAN_POINT ( 'NONE',  ( -3.712013335537174572E-16, -29.81250000000000000, -6.062177826491070398 ) ) ;
#5006=EDGE_CURVE ( 'NONE', #8385, #8014, #3595, .T. ) ;
#5008=CARTESIAN_POINT ( 'NONE',  ( -5.385316468750001029, -27.59895833299193413, -3.109213912904136734 ) ) ;
#5033=CARTESIAN_POINT ( 'NONE',  ( 5.385316468750001029, -27.50520833299193413, 3.109213912904134958 ) ) ;
#5040=CARTESIAN_POINT ( 'NONE',  ( 0.000000000000000000, -30.00000000000000000, -6.250000000000002665 ) ) ;
#5041=EDGE_CURVE ( 'NONE', #2851, #4496, #5724, .T. ) ;
#5045=CARTESIAN_POINT ( 'NONE',  ( 1.406733260263393293, -27.76116454900182973, -5.250000000000000000 ) ) ;
#5047=DIRECTION ( 'NONE',  ( 0.000000000000000000, -1.000000000000000000, 0.000000000000000000 ) ) ;
#5048=CARTESIAN_POINT ( 'NONE',  ( -3.807688866302469071E-16, -28.67187499965860198, -6.218427825808274356 ) ) ;
#5051=VECTOR ( 'NONE', #2878, 1000.000000000000000 ) ;
#5056=CARTESIAN_POINT ( 'NONE',  ( 5.385316468749999252, -27.18229166632526628, -3.109213912904139399 ) ) ;
#5058=CARTESIAN_POINT ( 'NONE',  ( -5.385316468749998364, -27.30729166632526983, 3.109213912904140287 ) ) ;
#5066=PRODUCT ( 'cone', 'cone', '', ( #4648 ) ) ;
#5069=FACE_OUTER_BOUND ( 'NONE', #743, .T. ) ;
#5070=CARTESIAN_POINT ( 'NONE',  ( -2.625000000000000444, -27.79166666666666430, -4.546633369868303021 ) ) ;
#5074=CARTESIAN_POINT ( 'NONE',  ( 5.250000000000000000, -28.06249999931720396, -6.429395695523604153E-16 ) ) ;
#5082=CARTESIAN_POINT ( 'NONE',  ( 1.142306659890740623E-15, -28.04687499965860198, 6.218427825808274356 ) ) ;
#5086=AXIS2_PLACEMENT_3D ( 'NONE', #7147, #7848, #9100 ) ;
#5087=ORIENTED_EDGE ( 'NONE', *, *, #761, .T. ) ;
#5088=CARTESIAN_POINT ( 'NONE',  ( -5.249999999999999112, -27.95833333265052900, -3.031088913245534755 ) ) ;
#5091=CARTESIAN_POINT ( 'NONE',  ( 1.142306659890740623E-15, -28.04687499965860198, 6.218427825808274356 ) ) ;
#5094=CYLINDRICAL_SURFACE ( 'NONE', #6574, 5.250000000000000000 ) ;
#5095=CARTESIAN_POINT ( 'NONE',  ( 2.161402558328724325E-14, -28.99999999931720751, -5.250000000000000000 ) ) ;
#5097=CARTESIAN_POINT ( 'NONE',  ( 0.000000000000000000, -27.00000000000000000, 0.000000000000000000 ) ) ;
#5099=CARTESIAN_POINT ( 'NONE',  ( -5.250000000000000000, -27.45833333265053611, -3.031088913245534755 ) ) ;
#5101=FACE_OUTER_BOUND ( 'NONE', #4794, .T. ) ;
#5105=CARTESIAN_POINT ( 'NONE',  ( -2.692658234374996518, -27.53645833299193413, 4.663820869356208654 ) ) ;
#5107=ORIENTED_EDGE ( 'NONE', *, *, #4861, .T. ) ;
#5108=CARTESIAN_POINT ( 'NONE',  ( 1.142306659890740623E-15, -27.26562499965860553, 6.218427825808274356 ) ) ;
#5112=EDGE_CURVE ( 'NONE', #6553, #7820, #3642, .T. ) ;
#5114=CARTESIAN_POINT ( 'NONE',  ( 5.250000000000000000, -27.35416666666666430, -3.031088913245536531 ) ) ;
#5118=CARTESIAN_POINT ( 'NONE',  ( 8.603239422292019767E-08, -29.99999999999999645, -5.249999999999998224 ) ) ;
#5122=ORIENTED_EDGE ( 'NONE', *, *, #6771, .F. ) ;
#5127=CARTESIAN_POINT ( 'NONE',  ( 0.000000000000000000, -27.00000000000000000, -6.250000000000000000 ) ) ;
#5128=CARTESIAN_POINT ( 'NONE',  ( 1.142306659890740623E-15, -27.79687499965860198, 6.218427825808274356 ) ) ;
#5131=CARTESIAN_POINT ( 'NONE',  ( 5.249999999999999112, -29.29166666598386826, -3.031088913245536975 ) ) ;
#5134=( BOUNDED_CURVE ( )  B_SPLINE_CURVE ( 2, ( #5663, #38, #4916, #8592, #7854, #2092, #1347, #7812, #7018 ),
 .UNSPECIFIED., .F., .F. ) 
 B_SPLINE_CURVE_WITH_KNOTS ( ( 3, 2, 2, 2, 3 ),
 ( 0.5208333333333333703, 0.5277777777777777901, 0.5416666666666666297, 0.5555555555555555802, 0.5625000000000000000 ),
 .UNSPECIFIED. ) 
 CURVE ( )  GEOMETRIC_REPRESENTATION_ITEM ( )  RATIONAL_B_SPLINE_CURVE ( ( 0.9330127018922192983, 0.9330127018922198534, 1.000000000000000000, 0.8660254037844387076, 1.000000000000000000, 0.8660254037844387076, 1.000000000000000000, 0.9330127018922194093, 0.9330127018922194093 ) ) 
 REPRESENTATION_ITEM ( '' )  );
#5136=CARTESIAN_POINT ( 'NONE',  ( -6.972266317189433020E-16, -29.81250000000000000, -5.250000000000000000 ) ) ;
#5138=CARTESIAN_POINT ( 'NONE',  ( 2.692658234375002735, -28.52604166632526628, 4.663820869356205101 ) ) ;
#5141=CARTESIAN_POINT ( 'NONE',  ( 2.692658234374998738, -27.41145833299193413, -4.663820869356206877 ) ) ;
#5145=DIRECTION ( 'NONE',  ( 0.000000000000000000, 0.000000000000000000, -1.000000000000000000 ) ) ;
#5147=CARTESIAN_POINT ( 'NONE',  ( -5.249999999999999112, -27.41666666598386826, 3.031088913245538308 ) ) ;
#5149=DIRECTION ( 'NONE',  ( 0.000000000000000000, -1.000000000000000000, 0.000000000000000000 ) ) ;
#5150=DIRECTION ( 'NONE',  ( 0.000000000000000000, 0.000000000000000000, -1.000000000000000000 ) ) ;
#5151=ORIENTED_EDGE ( 'NONE', *, *, #924, .T. ) ;
#5153=CARTESIAN_POINT ( 'NONE',  ( 1.142306659890740623E-15, -28.51562499965860198, 6.218427825808274356 ) ) ;
#5155=CARTESIAN_POINT ( 'NONE',  ( 0.000000000000000000, -27.00000000000000000, 0.000000000000000000 ) ) ;
#5157=CARTESIAN_POINT ( 'NONE',  ( -5.250000000000000000, -27.25000000000000000, 0.000000000000000000 ) ) ;
#5164=ADVANCED_FACE ( 'NONE', ( #4577 ), #1593, .F. ) ;
#5165=CARTESIAN_POINT ( 'NONE',  ( 5.250000000000000000, -27.37500000000000000, -6.429395695523604153E-16 ) ) ;
#5168=CARTESIAN_POINT ( 'NONE',  ( -5.249999999999999112, -29.95833333265053255, -3.031088913245534755 ) ) ;
#5177=ORIENTED_EDGE ( 'NONE', *, *, #2414, .F. ) ;
#5179=CARTESIAN_POINT ( 'NONE',  ( -5.385316468750001029, -28.13020833299193058, -3.109213912904136734 ) ) ;
#5182=VECTOR ( 'NONE', #1904, 1000.000000000000000 ) ;
#5186=CARTESIAN_POINT ( 'NONE',  ( -3.807688866302469071E-16, -28.17187499965860553, -6.218427825808274356 ) ) ;
#5190=CARTESIAN_POINT ( 'NONE',  ( -3.807688866302469071E-16, -27.39062499965860198, -6.218427825808274356 ) ) ;
#5196=CARTESIAN_POINT ( 'NONE',  ( 5.250000000000000888, -27.58333333265053966, 3.031088913245532979 ) ) ;
#5199=AXIS2_PLACEMENT_3D ( 'NONE', #8504, #4179, #1469 ) ;
#5200=CARTESIAN_POINT ( 'NONE',  ( 1.406733260263403507, -29.76116454900183328, -5.249999999999994671 ) ) ;
#5202=CARTESIAN_POINT ( 'NONE',  ( -5.385316468749998364, -27.80729166632526628, 3.109213912904140287 ) ) ;
#5206=CARTESIAN_POINT ( 'NONE',  ( 5.385316468749999252, -27.93229166632526628, -3.109213912904139399 ) ) ;
#5214=MANIFOLD_SOLID_BREP ( 'Thread1', #7124 ) ;
#5215=CARTESIAN_POINT ( 'NONE',  ( -2.624999999999996891, -30.14583333265053611, 4.546633369868304797 ) ) ;
#5220=( BOUNDED_CURVE ( )  B_SPLINE_CURVE ( 2, ( #1455, #6339, #6299, #7749, #4122, #2070, #5644, #4300, #1414 ),
 .UNSPECIFIED., .F., .T. ) 
 B_SPLINE_CURVE_WITH_KNOTS ( ( 3, 2, 2, 2, 3 ),
 ( 0.8125000000000000000, 0.8194444444444444198, 0.8333333333333333703, 0.8472222222222222099, 0.8541666666666667407 ),
 .UNSPECIFIED. ) 
 CURVE ( )  GEOMETRIC_REPRESENTATION_ITEM ( )  RATIONAL_B_SPLINE_CURVE ( ( 0.9330127018922194093, 0.9330127018922194093, 1.000000000000000000, 0.8660254037844387076, 1.000000000000000000, 0.8660254037844387076, 1.000000000000000000, 0.9330127018922187432, 0.9330127018922192983 ) ) 
 REPRESENTATION_ITEM ( '' )  );
#5226=CARTESIAN_POINT ( 'NONE',  ( 2.692658234374998738, -27.44270833299193413, -4.663820869356206877 ) ) ;
#5229=CARTESIAN_POINT ( 'NONE',  ( 2.692658234374998738, -27.94270833299193413, -4.663820869356206877 ) ) ;
#5234=CARTESIAN_POINT ( 'NONE',  ( 5.385316468750001029, -28.00520833299193413, 3.109213912904135846 ) ) ;
#5241=CONICAL_SURFACE ( 'NONE', #1840, 6.250000000000002665, 0.1221730476396033355 ) ;
#5242=CARTESIAN_POINT ( 'NONE',  ( 2.624999999999998668, -28.52083333265053611, -4.546633369868303021 ) ) ;
#5245=CARTESIAN_POINT ( 'NONE',  ( 5.249999999999999112, -29.54166666598386470, -3.031088913245536975 ) ) ;
#5246=CARTESIAN_POINT ( 'NONE',  ( 0.000000000000000000, -30.00000000000000000, 0.000000000000000000 ) ) ;
#5248=CARTESIAN_POINT ( 'NONE',  ( -5.385316468750000141, -27.82812499965860198, 0.000000000000000000 ) ) ;
#5252=CARTESIAN_POINT ( 'NONE',  ( -2.692658234375000514, -28.86979166632526983, -4.663820869356205989 ) ) ;
#5258=CARTESIAN_POINT ( 'NONE',  ( -2.625000000000000444, -27.29166666666666430, -4.546633369868303021 ) ) ;
#5264=CARTESIAN_POINT ( 'NONE',  ( 0.000000000000000000, -27.00000000000000000, 0.000000000000000000 ) ) ;
#5266=( LENGTH_UNIT ( ) NAMED_UNIT ( * ) SI_UNIT ( .MILLI., .METRE. ) );
#5273=CARTESIAN_POINT ( 'NONE',  ( -5.385316468750000141, -27.10937499965860198, 0.000000000000000000 ) ) ;
#5274=CARTESIAN_POINT ( 'NONE',  ( -5.385316468750001029, -28.88020833299193058, -3.109213912904136734 ) ) ;
#5277=CARTESIAN_POINT ( 'NONE',  ( -5.385316468750001029, -27.63020833299193413, -3.109213912904136734 ) ) ;
#5278=ORIENTED_EDGE ( 'NONE', *, *, #1228, .T. ) ;
#5279=CARTESIAN_POINT ( 'NONE',  ( 5.250000000000000888, -29.89583333333333215, 3.031088913245533423 ) ) ;
#5281=CARTESIAN_POINT ( 'NONE',  ( -5.385316468749998364, -27.33854166632526628, 3.109213912904140287 ) ) ;
#5282=VERTEX_POINT ( 'NONE', #6246 ) ;
#5283=CARTESIAN_POINT ( 'NONE',  ( -3.807688866302469071E-16, -28.64062499965860198, -6.218427825808274356 ) ) ;
#5286=CARTESIAN_POINT ( 'NONE',  ( 2.625000000000002220, -27.60416666598386826, 4.546633369868302132 ) ) ;
#5290=ORIENTED_EDGE ( 'NONE', *, *, #7150, .F. ) ;
#5291=CARTESIAN_POINT ( 'NONE',  ( 5.385316468750000141, -28.70312499965860198, -6.595110575850215044E-16 ) ) ;
#5295=CARTESIAN_POINT ( 'NONE',  ( -2.692658234375000514, -27.86979166632526628, -4.663820869356205989 ) ) ;
#5300=EDGE_CURVE ( 'NONE', #2431, #2212, #6030, .T. ) ;
#5302=CARTESIAN_POINT ( 'NONE',  ( 5.250000000000000000, -27.10416666666666430, -3.031088913245536531 ) ) ;
#5310=EDGE_CURVE ( 'NONE', #2524, #3224, #85, .T. ) ;
#5315=CARTESIAN_POINT ( 'NONE',  ( -3.807688866302469071E-16, -29.42187499965860198, -6.218427825808274356 ) ) ;
#5317=CARTESIAN_POINT ( 'NONE',  ( 2.692658234374998738, -29.69270833299193413, -4.663820869356206877 ) ) ;
#5318=VECTOR ( 'NONE', #7711, 1000.000000000000000 ) ;
#5323=CARTESIAN_POINT ( 'NONE',  ( 5.385316468750000141, -29.48437499965859843, -6.595110575850215044E-16 ) ) ;
#5326=CARTESIAN_POINT ( 'NONE',  ( -5.385316468750000141, -28.82812499965860198, 0.000000000000000000 ) ) ;
#5333=DIRECTION ( 'NONE',  ( 0.000000000000000000, 0.000000000000000000, -1.000000000000000000 ) ) ;
#5335=CYLINDRICAL_SURFACE ( 'NONE', #1481, 5.250000000000000000 ) ;
#5339=CARTESIAN_POINT ( 'NONE',  ( 5.385316468750001029, -29.22395833299193413, 3.109213912904135846 ) ) ;
#5342=CARTESIAN_POINT ( 'NONE',  ( 1.142306659890740623E-15, -28.26562499965860198, 6.218427825808274356 ) ) ;
#5350=CARTESIAN_POINT ( 'NONE',  ( 5.250000000000000000, -28.87499999999999645, -6.429395695523604153E-16 ) ) ;
#5365=CARTESIAN_POINT ( 'NONE',  ( -2.692658234375000514, -28.90104166632526983, -4.663820869356205989 ) ) ;
#5366=CARTESIAN_POINT ( 'NONE',  ( -3.807688866302469071E-16, -29.67187499965859487, -6.218427825808274356 ) ) ;
#5368=CARTESIAN_POINT ( 'NONE',  ( 2.692658234374998738, -29.94270833299193413, -4.663820869356206877 ) ) ;
#5370=ORIENTED_EDGE ( 'NONE', *, *, #173, .T. ) ;
#5373=CARTESIAN_POINT ( 'NONE',  ( 1.142306659890740623E-15, -29.29687499965860198, 6.218427825808274356 ) ) ;
#5374=ADVANCED_FACE ( 'NONE', ( #5545 ), #4842, .T. ) ;
#5376=CARTESIAN_POINT ( 'NONE',  ( -5.385316468750001029, -28.84895833299193413, -3.109213912904136734 ) ) ;
#5378=LINE ( 'NONE', #1203, #5182 ) ;
#5379=EDGE_CURVE ( 'NONE', #4857, #6768, #1973, .T. ) ;
#5381=CARTESIAN_POINT ( 'NONE',  ( 5.249999999999999112, -27.35416666666666430, -3.031088913245536975 ) ) ;
#5382=AXIS2_PLACEMENT_3D ( 'NONE', #7254, #2939, #4283 ) ;
#5386=CARTESIAN_POINT ( 'NONE',  ( 1.142306659890740623E-15, -30.01562499965860198, 6.218427825808274356 ) ) ;
#5388=CARTESIAN_POINT ( 'NONE',  ( 2.161402558328724325E-14, -29.56250000000000355, -5.250000000000000000 ) ) ;
#5389=CARTESIAN_POINT ( 'NONE',  ( -2.692658234374996518, -28.78645833299193413, 4.663820869356208654 ) ) ;
#5392=CARTESIAN_POINT ( 'NONE',  ( -5.249999999999997335, -30.16666666598387181, 3.031088913245538308 ) ) ;
#5397=ORIENTED_EDGE ( 'NONE', *, *, #645, .T. ) ;
#5398=CARTESIAN_POINT ( 'NONE',  ( -5.250000000000000000, -29.02083333333333570, -3.031088913245534755 ) ) ;
#5411=DIRECTION ( 'NONE',  ( 0.000000000000000000, -1.000000000000000000, 0.000000000000000000 ) ) ;
#5412=CARTESIAN_POINT ( 'NONE',  ( 2.692658234374998738, -28.94270833299193413, -4.663820869356206877 ) ) ;
#5413=CARTESIAN_POINT ( 'NONE',  ( -2.692658234374996518, -30.06770833299193413, 4.663820869356208654 ) ) ;
#5415=CARTESIAN_POINT ( 'NONE',  ( 5.385316468750000141, -29.23437499965859843, -6.595110575850215044E-16 ) ) ;
#5418=CARTESIAN_POINT ( 'NONE',  ( 1.406733260263390628, -28.42633545031536713, 5.250000000000001776 ) ) ;
#5420=CARTESIAN_POINT ( 'NONE',  ( 5.385316468750000141, -29.23437499965859843, -6.595110575850215044E-16 ) ) ;
#5423=CARTESIAN_POINT ( 'NONE',  ( 1.142306659890740623E-15, -28.51562499965860198, 6.218427825808274356 ) ) ;
#5426=ADVANCED_FACE ( 'NONE', ( #6325 ), #5241, .T. ) ;
#5430=EDGE_CURVE ( 'NONE', #6037, #2331, #5587, .T. ) ;
#5433=SHAPE_DEFINITION_REPRESENTATION ( #4989, #6994 ) ;
#5434=CARTESIAN_POINT ( 'NONE',  ( 2.692658234375002735, -29.74479166632526983, 4.663820869356205101 ) ) ;
#5436=CARTESIAN_POINT ( 'NONE',  ( -2.625000000000000444, -28.04166666666666785, -4.546633369868303021 ) ) ;
#5437=CARTESIAN_POINT ( 'NONE',  ( -5.385316468749998364, -30.05729166632526628, 3.109213912904140287 ) ) ;
#5439=EDGE_LOOP ( 'NONE', ( #2207, #1733, #8270, #7956 ) ) ;
#5444=ORIENTED_EDGE ( 'NONE', *, *, #5041, .T. ) ;
#5445=FILL_AREA_STYLE ('',( #3968 ) ) ;
#5446=CARTESIAN_POINT ( 'NONE',  ( -2.625000000000000444, -28.79166666666666785, -4.546633369868303021 ) ) ;
#5451=CARTESIAN_POINT ( 'NONE',  ( -9.180150650966086169E-15, -28.18749999999999645, 5.249999999999999112 ) ) ;
#5453=CARTESIAN_POINT ( 'NONE',  ( -1.406733260263402174, -29.13616454900182973, 5.249999999999995559 ) ) ;
#5458=MECHANICAL_DESIGN_GEOMETRIC_PRESENTATION_REPRESENTATION('',(#4272),#2053);
#5460=CARTESIAN_POINT ( 'NONE',  ( -2.692658234374996518, -29.06770833299193413, 4.663820869356208654 ) ) ;
#5462=CARTESIAN_POINT ( 'NONE',  ( -5.385316468749998364, -29.83854166632526628, 3.109213912904140287 ) ) ;
#5469=CARTESIAN_POINT ( 'NONE',  ( -2.692658234375000514, -29.90104166632526983, -4.663820869356205989 ) ) ;
#5471=CARTESIAN_POINT ( 'NONE',  ( -2.692658234375000514, -28.61979166632526628, -4.663820869356205989 ) ) ;
#5474=LINE ( 'NONE', #4223, #8493 ) ;
#5481=CARTESIAN_POINT ( 'NONE',  ( -2.692658234374996518, -29.53645833299193413, 4.663820869356208654 ) ) ;
#5483=ADVANCED_FACE ( 'NONE', ( #6286 ), #53, .F. ) ;
#5484=CARTESIAN_POINT ( 'NONE',  ( 5.249999999999999112, -28.54166666598386470, -3.031088913245536975 ) ) ;
#5485=CARTESIAN_POINT ( 'NONE',  ( 2.692658234374998738, -29.91145833299193413, -4.663820869356206877 ) ) ;
#5488=VECTOR ( 'NONE', #8452, 1000.000000000000000 ) ;
#5495=CARTESIAN_POINT ( 'NONE',  ( 5.250000000000000000, -27.87500000000000000, -6.429395695523604153E-16 ) ) ;
#5499=CARTESIAN_POINT ( 'NONE',  ( 1.406733260263398400, -28.07366454968463287, -5.249999999999997335 ) ) ;
#5509=CYLINDRICAL_SURFACE ( 'NONE', #7858, 5.250000000000000000 ) ;
#5510=CARTESIAN_POINT ( 'NONE',  ( -5.250000000000000000, -28.70833333265053611, -3.031088913245534755 ) ) ;
#5513=CARTESIAN_POINT ( 'NONE',  ( 5.385316468750001029, -29.75520833299193413, 3.109213912904135846 ) ) ;
#5519=CARTESIAN_POINT ( 'NONE',  ( 5.385316468750001029, -29.50520833299193413, 3.109213912904135846 ) ) ;
#5521=CARTESIAN_POINT ( 'NONE',  ( -2.692658234374996518, -29.53645833299193413, 4.663820869356208654 ) ) ;
#5527=DIRECTION ( 'NONE',  ( 0.000000000000000000, -1.000000000000000000, 0.000000000000000000 ) ) ;
#5532=CARTESIAN_POINT ( 'NONE',  ( 2.692658234374998738, -29.66145833299193413, -4.663820869356206877 ) ) ;
#5535=CARTESIAN_POINT ( 'NONE',  ( 2.692658234375002735, -29.99479166632526628, 4.663820869356205101 ) ) ;
#5537=CARTESIAN_POINT ( 'NONE',  ( 2.624999999999998668, -30.02083333265053611, -4.546633369868303021 ) ) ;
#5538=CYLINDRICAL_SURFACE ( 'NONE', #1351, 5.250000000000000000 ) ;
#5540=CARTESIAN_POINT ( 'NONE',  ( -2.625000000000000444, -28.04166666666666785, -4.546633369868303021 ) ) ;
#5545=FACE_OUTER_BOUND ( 'NONE', #585, .T. ) ;
#5550=FACE_OUTER_BOUND ( 'NONE', #8624, .T. ) ;
#5551=CARTESIAN_POINT ( 'NONE',  ( -5.250000000000000000, -29.43749999931720041, 0.000000000000000000 ) ) ;
#5559=CARTESIAN_POINT ( 'NONE',  ( -2.625000000000000444, -27.54166666666666430, -4.546633369868303021 ) ) ;
#5561=CARTESIAN_POINT ( 'NONE',  ( -2.692658234374996518, -30.06770833299193413, 4.663820869356208654 ) ) ;
#5562=EDGE_LOOP ( 'NONE', ( #2669, #6524, #8541, #4708 ) ) ;
#5563=CARTESIAN_POINT ( 'NONE',  ( 2.692658234375002735, -29.74479166632526983, 4.663820869356205101 ) ) ;
#5566=DIRECTION ( 'NONE',  ( -0.8660254037844402619, -0.4999999999999970579, 0.000000000000000000 ) ) ;
#5571=CARTESIAN_POINT ( 'NONE',  ( -1.406733260263389518, -28.23883544963256753, -5.250000000000001776 ) ) ;
#5575=( BOUNDED_CURVE ( )  B_SPLINE_CURVE ( 2, ( #6833, #9101, #3254, #5381, #3999, #1206, #8233, #1155, #458 ),
 .UNSPECIFIED., .F., .T. ) 
 B_SPLINE_CURVE_WITH_KNOTS ( ( 3, 2, 2, 2, 3 ),
 ( 0.1041666666666666713, 0.1111111111111111049, 0.1250000000000000000, 0.1388888888888888951, 0.1458333333333333426 ),
 .UNSPECIFIED. ) 
 CURVE ( )  GEOMETRIC_REPRESENTATION_ITEM ( )  RATIONAL_B_SPLINE_CURVE ( ( 0.9330127018922194093, 0.9330127018922194093, 1.000000000000000000, 0.8660254037844387076, 1.000000000000000000, 0.8660254037844387076, 1.000000000000000000, 0.9330127018922194093, 0.9330127018922194093 ) ) 
 REPRESENTATION_ITEM ( '' )  );
#5576=CARTESIAN_POINT ( 'NONE',  ( 5.385316468749999252, -29.93229166632526983, -3.109213912904139399 ) ) ;
#5583=CARTESIAN_POINT ( 'NONE',  ( -5.385316468750001029, -27.09895833299193413, -3.109213912904136734 ) ) ;
#5587=LINE ( 'NONE', #2104, #8656 ) ;
#5588=EDGE_CURVE ( 'NONE', #4395, #3470, #1996, .T. ) ;
#5590=LINE ( 'NONE', #7739, #2535 ) ;
#5592=DIRECTION ( 'NONE',  ( 0.000000000000000000, -1.000000000000000000, 0.000000000000000000 ) ) ;
#5593=CARTESIAN_POINT ( 'NONE',  ( 1.113604000661152470E-15, -29.37499999931719685, 6.062177826491070398 ) ) ;
#5594=CARTESIAN_POINT ( 'NONE',  ( 1.406733260263394847, -27.51116454900183683, -5.250000000000000000 ) ) ;
#5596=CARTESIAN_POINT ( 'NONE',  ( -1.406733260263393959, -27.23883544963257108, -5.250000000000000888 ) ) ;
#5600=CARTESIAN_POINT ( 'NONE',  ( 2.625000000000002220, -29.16666666666666785, 4.546633369868302132 ) ) ;
#5604=CARTESIAN_POINT ( 'NONE',  ( -5.385316468750001029, -29.09895833299193058, -3.109213912904136734 ) ) ;
#5616=CARTESIAN_POINT ( 'NONE',  ( 1.045839947578414884E-14, -28.24999999931720041, -5.249999999999999112 ) ) ;
#5617=CARTESIAN_POINT ( 'NONE',  ( 5.385316468749999252, -27.21354166632526628, -3.109213912904139399 ) ) ;
#5618=ADVANCED_FACE ( 'NONE', ( #4243, #3590 ), #2901, .F. ) ;
#5623=( BOUNDED_CURVE ( )  B_SPLINE_CURVE ( 2, ( #965, #8783, #4599, #2462, #1572, #3769, #4414, #1619, #8735 ),
 .UNSPECIFIED., .F., .T. ) 
 B_SPLINE_CURVE_WITH_KNOTS ( ( 3, 2, 2, 2, 3 ),
 ( 0.1458333333333333426, 0.1527777777777777901, 0.1666666666666666574, 0.1805555555555555525, 0.1875000000000000000 ),
 .UNSPECIFIED. ) 
 CURVE ( )  GEOMETRIC_REPRESENTATION_ITEM ( )  RATIONAL_B_SPLINE_CURVE ( ( 0.9330127018922194093, 0.9330127018922194093, 1.000000000000000000, 0.8660254037844387076, 1.000000000000000000, 0.8660254037844387076, 1.000000000000000000, 0.9330127018922194093, 0.9330127018922194093 ) ) 
 REPRESENTATION_ITEM ( '' )  );
#5624=CARTESIAN_POINT ( 'NONE',  ( -5.250000000000000000, -29.77083333333333570, -3.031088913245534755 ) ) ;
#5626=EDGE_CURVE ( 'NONE', #7281, #7319, #8591, .T. ) ;
#5630=DIRECTION ( 'NONE',  ( 0.000000000000000000, 0.000000000000000000, -1.000000000000000000 ) ) ;
#5636=CARTESIAN_POINT ( 'NONE',  ( -1.406733260263384411, -29.30133545031537068, -5.250000000000006217 ) ) ;
#5637=CARTESIAN_POINT ( 'NONE',  ( -2.624999999999996891, -29.14583333265053611, 4.546633369868304797 ) ) ;
#5644=CARTESIAN_POINT ( 'NONE',  ( -2.625000000000000444, -29.72916666598387181, -4.546633369868303021 ) ) ;
#5649=CARTESIAN_POINT ( 'NONE',  ( 2.692658234375002735, -29.49479166632526983, 4.663820869356205101 ) ) ;
#5656=CARTESIAN_POINT ( 'NONE',  ( 6.972266317189434006E-16, -27.24999999931720751, -5.250000000000000000 ) ) ;
#5663=CARTESIAN_POINT ( 'NONE',  ( 2.161402558328724325E-14, -28.56250000000000000, -5.250000000000000000 ) ) ;
#5664=CARTESIAN_POINT ( 'NONE',  ( -2.692658234374996518, -27.81770833299193413, 4.663820869356208654 ) ) ;
#5670=CARTESIAN_POINT ( 'NONE',  ( -5.249999999999999112, -29.22916666666666430, 3.031088913245538308 ) ) ;
#5676=AXIS2_PLACEMENT_3D ( 'NONE', #5246, #1718, #6685 ) ;
#5677=VECTOR ( 'NONE', #3426, 1000.000000000000000 ) ;
#5679=CARTESIAN_POINT ( 'NONE',  ( -5.250000000000000000, -28.95833333265053255, -3.031088913245534755 ) ) ;
#5686=AXIS2_PLACEMENT_3D ( 'NONE', #8710, #7461, #3792 ) ;
#5688=CARTESIAN_POINT ( 'NONE',  ( -5.250000000000000000, -28.93749999931720396, 0.000000000000000000 ) ) ;
#5690=ORIENTED_EDGE ( 'NONE', *, *, #97, .T. ) ;
#5691=AXIS2_PLACEMENT_3D ( 'NONE', #7075, #4884, #7736 ) ;
#5693=CARTESIAN_POINT ( 'NONE',  ( -5.385316468750001029, -29.59895833299193413, -3.109213912904136734 ) ) ;
#5697=CARTESIAN_POINT ( 'NONE',  ( -2.033577675846918216E-14, -29.93750000000000000, 5.250000000000000888 ) ) ;
#5706=CARTESIAN_POINT ( 'NONE',  ( 5.385316468749999252, -27.46354166632526983, -3.109213912904139399 ) ) ;
#5711=ORIENTED_EDGE ( 'NONE', *, *, #1617, .F. ) ;
#5713=CARTESIAN_POINT ( 'NONE',  ( -2.625000000000000444, -29.29166666666666785, -4.546633369868303021 ) ) ;
#5715=CARTESIAN_POINT ( 'NONE',  ( -5.385316468750000141, -27.57812499965860198, 0.000000000000000000 ) ) ;
#5719=CARTESIAN_POINT ( 'NONE',  ( 5.249999999999999112, -29.35416666666666430, -3.031088913245536975 ) ) ;
#5724=LINE ( 'NONE', #665, #1245 ) ;
#5725=DIRECTION ( 'NONE',  ( 0.000000000000000000, -1.000000000000000000, 0.000000000000000000 ) ) ;
#5726=DIRECTION ( 'NONE',  ( 0.000000000000000000, -1.000000000000000000, 0.000000000000000000 ) ) ;
#5731=DIRECTION ( 'NONE',  ( 0.000000000000000000, -1.000000000000000000, 0.000000000000000000 ) ) ;
#5733=( BOUNDED_CURVE ( )  B_SPLINE_CURVE ( 2, ( #916, #3764, #5892, #8686, #1712, #6635, #5799, #1665, #4596 ),
 .UNSPECIFIED., .F., .F. ) 
 B_SPLINE_CURVE_WITH_KNOTS ( ( 3, 2, 2, 2, 3 ),
 ( 0.06250000000000000000, 0.06944444444444444753, 0.08333333333333332871, 0.09722222222222222376, 0.1041666666666666713 ),
 .UNSPECIFIED. ) 
 CURVE ( )  GEOMETRIC_REPRESENTATION_ITEM ( )  RATIONAL_B_SPLINE_CURVE ( ( 0.9330127018922194093, 0.9330127018922194093, 1.000000000000000000, 0.8660254037844387076, 1.000000000000000000, 0.8660254037844387076, 1.000000000000000000, 0.9330127018922192983, 0.9330127018922194093 ) ) 
 REPRESENTATION_ITEM ( '' )  );
#5744=CARTESIAN_POINT ( 'NONE',  ( 2.625000000000002220, -27.35416666598386826, 4.546633369868302132 ) ) ;
#5746=CARTESIAN_POINT ( 'NONE',  ( 0.000000000000000000, -27.00000000000000000, 0.000000000000000000 ) ) ;
#5752=CARTESIAN_POINT ( 'NONE',  ( -3.807688866302469071E-16, -28.42187499965859843, -6.218427825808274356 ) ) ;
#5758=CARTESIAN_POINT ( 'NONE',  ( 5.250000000000000000, -29.62500000000000000, -6.429395695523604153E-16 ) ) ;
#5759=ORIENTED_EDGE ( 'NONE', *, *, #546, .F. ) ;
#5760=CARTESIAN_POINT ( 'NONE',  ( -5.385316468750000141, -27.07812499965860198, 0.000000000000000000 ) ) ;
#5770=DIRECTION ( 'NONE',  ( 0.8660254037844402619, -0.4999999999999970579, 0.000000000000000000 ) ) ;
#5780=ORIENTED_EDGE ( 'NONE', *, *, #6043, .T. ) ;
#5786=FACE_OUTER_BOUND ( 'NONE', #8623, .T. ) ;
#5788=AXIS2_PLACEMENT_3D ( 'NONE', #3441, #7528, #2040 ) ;
#5795=CARTESIAN_POINT ( 'NONE',  ( 0.000000000000000000, -27.00000000000000000, 0.000000000000000000 ) ) ;
#5796=CIRCLE ( 'NONE', #1800, 3.794308781941904574 ) ;
#5799=CARTESIAN_POINT ( 'NONE',  ( -2.625000000000000444, -27.47916666598386826, -4.546633369868303021 ) ) ;
#5802=CARTESIAN_POINT ( 'NONE',  ( 2.625000000000002220, -28.35416666598386826, 4.546633369868302132 ) ) ;
#5803=AXIS2_PLACEMENT_3D ( 'NONE', #3350, #551, #6180 ) ;
#5809=CARTESIAN_POINT ( 'NONE',  ( 5.385316468750001029, -28.72395833299193413, 3.109213912904135846 ) ) ;
#5810=CARTESIAN_POINT ( 'NONE',  ( 1.975475456537005874E-15, -28.68749999999999645, 5.250000000000000000 ) ) ;
#5811=EDGE_LOOP ( 'NONE', ( #1757, #4853, #6362, #8676 ) ) ;
#5812=CARTESIAN_POINT ( 'NONE',  ( -2.692658234374996518, -27.28645833299193413, 4.663820869356208654 ) ) ;
#5823=CARTESIAN_POINT ( 'NONE',  ( 1.045839947578414884E-14, -28.06249999999999289, -5.249999999999999112 ) ) ;
#5834=CARTESIAN_POINT ( 'NONE',  ( -5.385316468750001029, -27.63020833299193768, -3.109213912904136734 ) ) ;
#5841=CARTESIAN_POINT ( 'NONE',  ( 2.692658234374998738, -28.19270833299193413, -4.663820869356206877 ) ) ;
#5846=CYLINDRICAL_SURFACE ( 'NONE', #1620, 5.250000000000000000 ) ;
#5849=CARTESIAN_POINT ( 'NONE',  ( -2.624999999999996891, -28.39583333265053611, 4.546633369868304797 ) ) ;
#5854=CARTESIAN_POINT ( 'NONE',  ( 2.692658234374998738, -27.66145833299193413, -4.663820869356206877 ) ) ;
#5857=ORIENTED_EDGE ( 'NONE', *, *, #2944, .F. ) ;
#5858=CARTESIAN_POINT ( 'NONE',  ( 2.692658234374998738, -27.41145833299193413, -4.663820869356206877 ) ) ;
#5874=CARTESIAN_POINT ( 'NONE',  ( 5.249999999999999112, -27.10416666666666430, -3.031088913245536975 ) ) ;
#5877=ORIENTED_EDGE ( 'NONE', *, *, #6896, .T. ) ;
#5878=ADVANCED_FACE ( 'NONE', ( #377 ), #1639, .T. ) ;
#5879=CARTESIAN_POINT ( 'NONE',  ( -5.250000000000000000, -29.75000000000000000, 0.000000000000000000 ) ) ;
#5880=CARTESIAN_POINT ( 'NONE',  ( 2.692658234375002735, -28.02604166632526628, 4.663820869356205101 ) ) ;
#5886=CARTESIAN_POINT ( 'NONE',  ( 2.692658234375002735, -28.02604166632526628, 4.663820869356205101 ) ) ;
#5889=CARTESIAN_POINT ( 'NONE',  ( 5.250000000000000888, -28.83333333265053966, 3.031088913245533423 ) ) ;
#5892=CARTESIAN_POINT ( 'NONE',  ( -2.624999999999996891, -27.39583333265053611, 4.546633369868304797 ) ) ;
#5894=CARTESIAN_POINT ( 'NONE',  ( -3.712013335537174572E-16, -28.24999999931720041, -6.062177826491070398 ) ) ;
#5899=CARTESIAN_POINT ( 'NONE',  ( 2.692658234374998738, -28.41145833299193413, -4.663820869356206877 ) ) ;
#5904=CARTESIAN_POINT ( 'NONE',  ( -2.692658234375000514, -27.36979166632526628, -4.663820869356205989 ) ) ;
#5906=EDGE_LOOP ( 'NONE', ( #5122, #1727, #3834, #1026 ) ) ;
#5912=CARTESIAN_POINT ( 'NONE',  ( -5.249999999999999112, -29.91666666598387181, 3.031088913245538308 ) ) ;
#5915=LINE ( 'NONE', #3144, #1524 ) ;
#5919=CARTESIAN_POINT ( 'NONE',  ( -5.250000000000000000, -30.00000000000000000, 0.000000000000000000 ) ) ;
#5924=( BOUNDED_CURVE ( )  B_SPLINE_CURVE ( 2, ( #106, #374, #4392, #5874, #3919, #846, #3694, #3005, #8667 ),
 .UNSPECIFIED., .F., .F. ) 
 B_SPLINE_CURVE_WITH_KNOTS ( ( 3, 2, 2, 2, 3 ),
 ( 0.02083333333333333218, 0.02777777777777777624, 0.04166666666666666435, 0.05555555555555555247, 0.06250000000000000000 ),
 .UNSPECIFIED. ) 
 CURVE ( )  GEOMETRIC_REPRESENTATION_ITEM ( )  RATIONAL_B_SPLINE_CURVE ( ( 0.9330127018922194093, 0.9330127018922194093, 1.000000000000000000, 0.8660254037844387076, 1.000000000000000000, 0.8660254037844387076, 1.000000000000000000, 0.9330127018922194093, 0.9330127018922194093 ) ) 
 REPRESENTATION_ITEM ( '' )  );
#5929=CARTESIAN_POINT ( 'NONE',  ( 5.385316468750001029, -27.75520833299194123, 3.109213912904135846 ) ) ;
#5933=CARTESIAN_POINT ( 'NONE',  ( 5.385316468750000141, -28.23437499965860198, -6.595110575850215044E-16 ) ) ;
#5940=CARTESIAN_POINT ( 'NONE',  ( 5.250000000000000888, -28.08333333265053255, 3.031088913245532979 ) ) ;
#5944=EDGE_CURVE ( 'NONE', #7114, #3963, #1291, .T. ) ;
#5948=CARTESIAN_POINT ( 'NONE',  ( -5.385316468749998364, -27.55729166632526628, 3.109213912904140287 ) ) ;
#5950=CARTESIAN_POINT ( 'NONE',  ( -2.625000000000000444, -28.54166666666666785, -4.546633369868303021 ) ) ;
#5952=CARTESIAN_POINT ( 'NONE',  ( 2.692658234375002735, -28.99479166632526983, 4.663820869356205101 ) ) ;
#5954=ORIENTED_EDGE ( 'NONE', *, *, #5588, .T. ) ;
#5959=CARTESIAN_POINT ( 'NONE',  ( -2.624999999999996891, -27.70833333333333215, 4.546633369868304797 ) ) ;
#5969=DIRECTION ( 'NONE',  ( 0.000000000000000000, 0.000000000000000000, -1.000000000000000000 ) ) ;
#5970=CARTESIAN_POINT ( 'NONE',  ( -3.807688866302469071E-16, -27.17187499965860198, -6.218427825808274356 ) ) ;
#5972=CARTESIAN_POINT ( 'NONE',  ( 2.692658234375002735, -27.52604166632526628, 4.663820869356205101 ) ) ;
#5973=ORIENTED_EDGE ( 'NONE', *, *, #6142, .T. ) ;
#5974=DIRECTION ( 'NONE',  ( -1.492469013153037857E-17, 0.9925461516413219831, 0.1218693434051477398 ) ) ;
#5976=CARTESIAN_POINT ( 'NONE',  ( 2.692658234374998738, -28.44270833299193413, -4.663820869356206877 ) ) ;
#5978=CIRCLE ( 'NONE', #1984, 6.250000000000000000 ) ;
#5982=CARTESIAN_POINT ( 'NONE',  ( -2.624999999999996891, -29.39583333265053611, 4.546633369868304797 ) ) ;
#5985=CARTESIAN_POINT ( 'NONE',  ( 5.250000000000000000, -28.56249999931720396, -6.429395695523604153E-16 ) ) ;
#5988=EDGE_CURVE ( 'NONE', #8128, #8745, #3252, .T. ) ;
#5989=CARTESIAN_POINT ( 'NONE',  ( 5.250000000000000000, -29.56249999931720041, -6.429395695523604153E-16 ) ) ;
#5990=ORIENTED_EDGE ( 'NONE', *, *, #4524, .F. ) ;
#5992=CARTESIAN_POINT ( 'NONE',  ( 5.385316468750001029, -28.22395833299193058, 3.109213912904135846 ) ) ;
#5996=CARTESIAN_POINT ( 'NONE',  ( 5.385316468750000141, -28.20312499965860198, -6.595110575850215044E-16 ) ) ;
#5998=ORIENTED_EDGE ( 'NONE', *, *, #4871, .F. ) ;
#6003=CARTESIAN_POINT ( 'NONE',  ( -2.624999999999996891, -27.45833333333333570, 4.546633369868304797 ) ) ;
#6016=CARTESIAN_POINT ( 'NONE',  ( 2.692658234374998738, -28.44270833299193413, -4.663820869356206877 ) ) ;
#6019=CARTESIAN_POINT ( 'NONE',  ( -5.385316468749998364, -29.08854166632526628, 3.109213912904140287 ) ) ;
#6021=CARTESIAN_POINT ( 'NONE',  ( 2.624999999999998668, -28.33333333333333215, -4.546633369868303021 ) ) ;
#6023=CARTESIAN_POINT ( 'NONE',  ( 5.385316468749999252, -28.21354166632526983, -3.109213912904139399 ) ) ;
#6025=CARTESIAN_POINT ( 'NONE',  ( -5.385316468749998364, -28.30729166632526628, 3.109213912904140287 ) ) ;
#6030=( BOUNDED_CURVE ( )  B_SPLINE_CURVE ( 2, ( #3976, #5453, #480, #6106, #6805, #429, #1837, #3371, #8299 ),
 .UNSPECIFIED., .F., .F. ) 
 B_SPLINE_CURVE_WITH_KNOTS ( ( 3, 2, 2, 2, 3 ),
 ( 0.6458333333333333703, 0.6527777777777777901, 0.6666666666666666297, 0.6805555555555555802, 0.6875000000000000000 ),
 .UNSPECIFIED. ) 
 CURVE ( )  GEOMETRIC_REPRESENTATION_ITEM ( )  RATIONAL_B_SPLINE_CURVE ( ( 0.9330127018922192983, 0.9330127018922198534, 1.000000000000000000, 0.8660254037844387076, 1.000000000000000000, 0.8660254037844387076, 1.000000000000000000, 0.9330127018922194093, 0.9330127018922194093 ) ) 
 REPRESENTATION_ITEM ( '' )  );
#6032=EDGE_LOOP ( 'NONE', ( #8803, #5990, #2899, #5690 ) ) ;
#6034=CARTESIAN_POINT ( 'NONE',  ( -2.692658234375000514, -29.11979166632526983, -4.663820869356205989 ) ) ;
#6037=VERTEX_POINT ( 'NONE', #7716 ) ;
#6038=CARTESIAN_POINT ( 'NONE',  ( 5.385316468749999252, -28.43229166632526983, -3.109213912904139399 ) ) ;
#6043=EDGE_CURVE ( 'NONE', #4503, #8948, #7035, .T. ) ;
#6047=CARTESIAN_POINT ( 'NONE',  ( 1.113604000661152470E-15, -27.18750000000000000, 6.062177826491070398 ) ) ;
#6062=CARTESIAN_POINT ( 'NONE',  ( -5.385316468750001029, -28.63020833299193413, -3.109213912904136734 ) ) ;
#6063=CARTESIAN_POINT ( 'NONE',  ( 1.142306659890740623E-15, -30.04687499965859487, 6.218427825808274356 ) ) ;
#6065=CARTESIAN_POINT ( 'NONE',  ( -3.807688866302469071E-16, -29.67187499965860198, -6.218427825808274356 ) ) ;
#6070=CARTESIAN_POINT ( 'NONE',  ( -2.692658234374996518, -29.56770833299193413, 4.663820869356208654 ) ) ;
#6072=CARTESIAN_POINT ( 'NONE',  ( -5.385316468750000141, -28.32812499965860198, 0.000000000000000000 ) ) ;
#6089=CARTESIAN_POINT ( 'NONE',  ( 5.385316468749999252, -28.68229166632526983, -3.109213912904139399 ) ) ;
#6095=( BOUNDED_CURVE ( )  B_SPLINE_CURVE ( 2, ( #1737, #4573, #8691, #5245, #5989, #2415, #3722, #7907, #3030 ),
 .UNSPECIFIED., .F., .F. ) 
 B_SPLINE_CURVE_WITH_KNOTS ( ( 3, 2, 2, 2, 3 ),
 ( 0.7708333333333333703, 0.7777777777777777901, 0.7916666666666666297, 0.8055555555555555802, 0.8125000000000000000 ),
 .UNSPECIFIED. ) 
 CURVE ( )  GEOMETRIC_REPRESENTATION_ITEM ( )  RATIONAL_B_SPLINE_CURVE ( ( 0.9330127018922192983, 0.9330127018922198534, 1.000000000000000000, 0.8660254037844387076, 1.000000000000000000, 0.8660254037844387076, 1.000000000000000000, 0.9330127018922194093, 0.9330127018922194093 ) ) 
 REPRESENTATION_ITEM ( '' )  );
#6097=ORIENTED_EDGE ( 'NONE', *, *, #851, .F. ) ;
#6099=CARTESIAN_POINT ( 'NONE',  ( -5.250000000000000000, -28.99999999999999645, 0.000000000000000000 ) ) ;
#6106=CARTESIAN_POINT ( 'NONE',  ( -5.249999999999997335, -29.16666666598386826, 3.031088913245538308 ) ) ;
#6115=CARTESIAN_POINT ( 'NONE',  ( 5.385316468749999252, -28.96354166632526983, -3.109213912904138954 ) ) ;
#6117=CARTESIAN_POINT ( 'NONE',  ( -5.385316468749998364, -28.83854166632526628, 3.109213912904140287 ) ) ;
#6123=CARTESIAN_POINT ( 'NONE',  ( 5.385316468749999252, -28.71354166632526628, -3.109213912904139399 ) ) ;
#6125=CARTESIAN_POINT ( 'NONE',  ( 5.385316468749999252, -28.18229166632526628, -3.109213912904138954 ) ) ;
#6127=FACE_OUTER_BOUND ( 'NONE', #4418, .T. ) ;
#6136=CARTESIAN_POINT ( 'NONE',  ( -2.692658234375000514, -28.86979166632526983, -4.663820869356205989 ) ) ;
#6141=CARTESIAN_POINT ( 'NONE',  ( 1.142306659890740623E-15, -29.01562499965860198, 6.218427825808274356 ) ) ;
#6142=EDGE_CURVE ( 'NONE', #3963, #8099, #4146, .T. ) ;
#6150=PRESENTATION_STYLE_ASSIGNMENT (( #7545 ) ) ;
#6151=CARTESIAN_POINT ( 'NONE',  ( -2.624999999999996891, -27.95833333333333215, 4.546633369868304797 ) ) ;
#6152=ORIENTED_EDGE ( 'NONE', *, *, #1197, .F. ) ;
#6158=( BOUNDED_CURVE ( )  B_SPLINE_CURVE ( 2, ( #3840, #8672, #2919, #809, #3652, #6477, #7974, #2961, #112 ),
 .UNSPECIFIED., .F., .F. ) 
 B_SPLINE_CURVE_WITH_KNOTS ( ( 3, 2, 2, 2, 3 ),
 ( 0.8541666666666667407, 0.8611111111111111605, 0.8750000000000000000, 0.8888888888888888395, 0.8958333333333333703 ),
 .UNSPECIFIED. ) 
 CURVE ( )  GEOMETRIC_REPRESENTATION_ITEM ( )  RATIONAL_B_SPLINE_CURVE ( ( 0.9330127018922192983, 0.9330127018922198534, 1.000000000000000000, 0.8660254037844387076, 1.000000000000000000, 0.8660254037844387076, 1.000000000000000000, 0.9330127018922187432, 0.9330127018922192983 ) ) 
 REPRESENTATION_ITEM ( '' )  );
#6159=LINE ( 'NONE', #9115, #3721 ) ;
#6164=CARTESIAN_POINT ( 'NONE',  ( 5.385316468750001029, -28.75520833299193413, 3.109213912904134958 ) ) ;
#6166=FACE_OUTER_BOUND ( 'NONE', #4391, .T. ) ;
#6167=CARTESIAN_POINT ( 'NONE',  ( -2.692658234375000514, -29.15104166632526983, -4.663820869356205989 ) ) ;
#6173=CARTESIAN_POINT ( 'NONE',  ( 5.385316468750001029, -29.25520833299193058, 3.109213912904135846 ) ) ;
#6175=VERTEX_POINT ( 'NONE', #5095 ) ;
#6176=CARTESIAN_POINT ( 'NONE',  ( -5.385316468750001029, -28.59895833299193413, -3.109213912904136734 ) ) ;
#6179=( BOUNDED_CURVE ( )  B_SPLINE_CURVE ( 2, ( #4850, #2819, #7696, #5596, #1321 ),
 .UNSPECIFIED., .F., .T. ) 
 B_SPLINE_CURVE_WITH_KNOTS ( ( 3, 2, 3 ),
 ( 0.000000000000000000, 0.01388888888888888985, 0.02083333333333333565 ),
 .UNSPECIFIED. ) 
 CURVE ( )  GEOMETRIC_REPRESENTATION_ITEM ( )  RATIONAL_B_SPLINE_CURVE ( ( 1.000000000000000000, 0.8660254037844387076, 1.000000000000000000, 0.9330127018922192983, 0.9330127018922194093 ) ) 
 REPRESENTATION_ITEM ( '' )  );
#6180=DIRECTION ( 'NONE',  ( 1.000000000000000000, 0.000000000000000000, 0.000000000000000000 ) ) ;
#6181=FACE_OUTER_BOUND ( 'NONE', #6917, .T. ) ;
#6184=DIRECTION ( 'NONE',  ( 0.000000000000000000, -1.000000000000000000, 0.000000000000000000 ) ) ;
#6186=CARTESIAN_POINT ( 'NONE',  ( 2.692658234374998738, -29.41145833299193413, -4.663820869356206877 ) ) ;
#6188=CARTESIAN_POINT ( 'NONE',  ( 1.975475456537005874E-15, -27.93749999999999289, 5.250000000000000000 ) ) ;
#6189=CARTESIAN_POINT ( 'NONE',  ( -5.385316468750001029, -29.59895833299193413, -3.109213912904136734 ) ) ;
#6191=ORIENTED_EDGE ( 'NONE', *, *, #2736, .T. ) ;
#6197=CARTESIAN_POINT ( 'NONE',  ( 2.624999999999998668, -28.08333333333333215, -4.546633369868303021 ) ) ;
#6207=CARTESIAN_POINT ( 'NONE',  ( -2.033577675846918216E-14, -29.18750000000000355, 5.250000000000000888 ) ) ;
#6208=EDGE_CURVE ( 'NONE', #3979, #2331, #2902, .T. ) ;
#6209=CARTESIAN_POINT ( 'NONE',  ( 5.250000000000000000, -29.04166666598387181, -3.031088913245536531 ) ) ;
#6210=CARTESIAN_POINT ( 'NONE',  ( -2.692658234374996518, -29.81770833299193413, 4.663820869356208654 ) ) ;
#6212=CARTESIAN_POINT ( 'NONE',  ( -5.385316468749998364, -29.33854166632526983, 3.109213912904140287 ) ) ;
#6218=CARTESIAN_POINT ( 'NONE',  ( -5.385316468750000141, -29.10937499965859843, 0.000000000000000000 ) ) ;
#6219=ORIENTED_EDGE ( 'NONE', *, *, #6789, .F. ) ;
#6220=CARTESIAN_POINT ( 'NONE',  ( 2.692658234374998738, -27.91145833299193413, -4.663820869356206877 ) ) ;
#6222=DIRECTION ( 'NONE',  ( -0.000000000000000000, 1.000000000000000000, -0.000000000000000000 ) ) ;
#6223=CARTESIAN_POINT ( 'NONE',  ( -9.180150650966086169E-15, -28.43750000000000000, 5.249999999999999112 ) ) ;
#6224=CARTESIAN_POINT ( 'NONE',  ( 0.000000000000000000, -27.00000000000000000, 0.000000000000000000 ) ) ;
#6230=CARTESIAN_POINT ( 'NONE',  ( 2.692658234374998738, -29.16145833299193413, -4.663820869356206877 ) ) ;
#6233=( BOUNDED_CURVE ( )  B_SPLINE_CURVE ( 2, ( #8183, #8370, #8962, #4047, #6879, #2611, #360, #8275, #1908 ),
 .UNSPECIFIED., .F., .F. ) 
 B_SPLINE_CURVE_WITH_KNOTS ( ( 3, 2, 2, 2, 3 ),
 ( 0.3958333333333333703, 0.4027777777777777901, 0.4166666666666666852, 0.4305555555555555802, 0.4375000000000000000 ),
 .UNSPECIFIED. ) 
 CURVE ( )  GEOMETRIC_REPRESENTATION_ITEM ( )  RATIONAL_B_SPLINE_CURVE ( ( 0.9330127018922194093, 0.9330127018922196314, 1.000000000000000000, 0.8660254037844387076, 1.000000000000000000, 0.8660254037844387076, 1.000000000000000000, 0.9330127018922194093, 0.9330127018922194093 ) ) 
 REPRESENTATION_ITEM ( '' )  );
#6234=CARTESIAN_POINT ( 'NONE',  ( 5.385316468749999252, -29.43229166632526983, -3.109213912904139399 ) ) ;
#6238=ADVANCED_FACE ( 'NONE', ( #7050 ), #2165, .F. ) ;
#6240=CARTESIAN_POINT ( 'NONE',  ( 5.250000000000000888, -27.89583333333332860, 3.031088913245532979 ) ) ;
#6243=DIRECTION ( 'NONE',  ( 0.000000000000000000, -1.000000000000000000, 0.000000000000000000 ) ) ;
#6246=CARTESIAN_POINT ( 'NONE',  ( 8.603239422292021091E-08, -29.99999999999999645, -5.249999999999998224 ) ) ;
#6251=CARTESIAN_POINT ( 'NONE',  ( -2.033577675846918216E-14, -29.68750000000000355, 5.250000000000000888 ) ) ;
#6252=CARTESIAN_POINT ( 'NONE',  ( 5.250000000000000888, -29.33333333265053255, 3.031088913245532979 ) ) ;
#6253=CARTESIAN_POINT ( 'NONE',  ( -5.385316468750000141, -30.10937499965859843, 0.000000000000000000 ) ) ;
#6260=CARTESIAN_POINT ( 'NONE',  ( -2.033577675846918216E-14, -29.18750000000000355, 5.250000000000000888 ) ) ;
#6262=CARTESIAN_POINT ( 'NONE',  ( -5.250000000000000000, -27.20833333265053966, -3.031088913245534755 ) ) ;
#6264=CARTESIAN_POINT ( 'NONE',  ( -5.385316468750000141, -29.32812499965859843, 0.000000000000000000 ) ) ;
#6267=DIRECTION ( 'NONE',  ( 0.000000000000000000, -1.000000000000000000, 0.000000000000000000 ) ) ;
#6268=CARTESIAN_POINT ( 'NONE',  ( 0.000000000000000000, -27.00000000000000000, -5.250000000000000000 ) ) ;
#6270=CARTESIAN_POINT ( 'NONE',  ( 5.250000000000000888, -28.33333333265052900, 3.031088913245533423 ) ) ;
#6271=CARTESIAN_POINT ( 'NONE',  ( 2.625000000000002220, -27.85416666598386826, 4.546633369868302132 ) ) ;
#6273=CARTESIAN_POINT ( 'NONE',  ( -1.406733260263389518, -28.05133545031536357, -5.250000000000001776 ) ) ;
#6274=CARTESIAN_POINT ( 'NONE',  ( -5.385316468750000141, -29.57812499965859843, 0.000000000000000000 ) ) ;
#6281=CARTESIAN_POINT ( 'NONE',  ( -2.624999999999996891, -28.20833333333333215, 4.546633369868304797 ) ) ;
#6286=FACE_OUTER_BOUND ( 'NONE', #6701, .T. ) ;
#6291=CARTESIAN_POINT ( 'NONE',  ( -1.406733260263391960, -28.69866454968462577, 5.250000000000000000 ) ) ;
#6292=CARTESIAN_POINT ( 'NONE',  ( 1.113604000661152470E-15, -29.62499999931720041, 6.062177826491070398 ) ) ;
#6299=CARTESIAN_POINT ( 'NONE',  ( -2.624999999999996891, -29.64583333265053611, 4.546633369868304797 ) ) ;
#6301=EDGE_CURVE ( 'NONE', #3979, #6553, #7277, .T. ) ;
#6303=CARTESIAN_POINT ( 'NONE',  ( 5.385316468750001029, -29.72395833299193413, 3.109213912904134958 ) ) ;
#6306=DIRECTION ( 'NONE',  ( 0.000000000000000000, 0.000000000000000000, -1.000000000000000000 ) ) ;
#6308=CARTESIAN_POINT ( 'NONE',  ( 5.249999999999999112, -28.85416666666667140, -3.031088913245536975 ) ) ;
#6312=CARTESIAN_POINT ( 'NONE',  ( -6.972266317189433020E-16, -27.74999999931720041, -5.250000000000000000 ) ) ;
#6315=CARTESIAN_POINT ( 'NONE',  ( 1.142306659890740623E-15, -30.01562499965860198, 6.218427825808274356 ) ) ;
#6317=CARTESIAN_POINT ( 'NONE',  ( -7.654042494670960565E-16, -30.00000000000000000, 6.250000000000002665 ) ) ;
#6320=CARTESIAN_POINT ( 'NONE',  ( 1.113604000661152470E-15, -29.68750000000000000, 6.062177826491070398 ) ) ;
#6325=FACE_OUTER_BOUND ( 'NONE', #2379, .T. ) ;
#6330=CARTESIAN_POINT ( 'NONE',  ( -2.625000000000000444, -28.79166666666666785, -4.546633369868303021 ) ) ;
#6331=CARTESIAN_POINT ( 'NONE',  ( -5.249999999999999112, -29.16666666598387181, 3.031088913245538308 ) ) ;
#6332=LINE ( 'NONE', #2109, #2424 ) ;
#6334=CARTESIAN_POINT ( 'NONE',  ( -5.385316468750000141, -30.10937499965859843, 0.000000000000000000 ) ) ;
#6337=EDGE_CURVE ( 'NONE', #6768, #6698, #6746, .T. ) ;
#6338=ORIENTED_EDGE ( 'NONE', *, *, #97, .F. ) ;
#6339=CARTESIAN_POINT ( 'NONE',  ( -1.406733260263391960, -29.63616454900182973, 5.250000000000000000 ) ) ;
#6343=VERTEX_POINT ( 'NONE', #5127 ) ;
#6344=CARTESIAN_POINT ( 'NONE',  ( -3.807688866302469071E-16, -29.64062499965859843, -6.218427825808274356 ) ) ;
#6350=DIRECTION ( 'NONE',  ( 0.000000000000000000, 0.9925461516413219831, -0.1218693434051477398 ) ) ;
#6351=CARTESIAN_POINT ( 'NONE',  ( -5.385316468750001029, -27.13020833299193413, -3.109213912904136734 ) ) ;
#6357=CARTESIAN_POINT ( 'NONE',  ( -2.692658234375000514, -28.40104166632526628, -4.663820869356205989 ) ) ;
#6360=VECTOR ( 'NONE', #6932, 1000.000000000000000 ) ;
#6362=ORIENTED_EDGE ( 'NONE', *, *, #4871, .T. ) ;
#6363=CARTESIAN_POINT ( 'NONE',  ( -5.250000000000000000, -29.52083333333333215, -3.031088913245534755 ) ) ;
#6364=CIRCLE ( 'NONE', #7571, 5.242490174541154069 ) ;
#6368=CARTESIAN_POINT ( 'NONE',  ( 1.406733260263403507, -29.32366454968462932, -5.249999999999994671 ) ) ;
#6373=CARTESIAN_POINT ( 'NONE',  ( -2.625000000000000444, -28.97916666598386826, -4.546633369868303021 ) ) ;
#6379=EDGE_CURVE ( 'NONE', #7379, #6698, #6621, .T. ) ;
#6394=LINE ( 'NONE', #29, #5051 ) ;
#6396=CARTESIAN_POINT ( 'NONE',  ( 2.692658234374998738, -27.19270833299193413, -4.663820869356206877 ) ) ;
#6403=CARTESIAN_POINT ( 'NONE',  ( 5.385316468750000141, -28.48437499965860198, -6.595110575850215044E-16 ) ) ;
#6408=CARTESIAN_POINT ( 'NONE',  ( 2.692658234374998738, -27.41145833299193413, -4.663820869356206877 ) ) ;
#6410=CARTESIAN_POINT ( 'NONE',  ( -2.692658234374996518, -27.53645833299193413, 4.663820869356208654 ) ) ;
#6420=CARTESIAN_POINT ( 'NONE',  ( 0.000000000000000000, -27.00000000000000000, 0.000000000000000000 ) ) ;
#6422=VECTOR ( 'NONE', #3440, 1000.000000000000000 ) ;
#6424=DIRECTION ( 'NONE',  ( 0.000000000000000000, 0.9925461516413219831, -0.1218693434051477398 ) ) ;
#6427=CARTESIAN_POINT ( 'NONE',  ( 5.250000000000000888, -28.08333333265053255, 3.031088913245533423 ) ) ;
#6428=CARTESIAN_POINT ( 'NONE',  ( -1.406733260263391960, -28.88616454900183328, 5.250000000000000000 ) ) ;
#6433=DIRECTION ( 'NONE',  ( 0.000000000000000000, 0.000000000000000000, -1.000000000000000000 ) ) ;
#6437=( BOUNDED_CURVE ( )  B_SPLINE_CURVE ( 2, ( #8766, #113, #7227, #5970, #8674, #854, #3653, #3010, #2209, #8070, #7936, #2397, #6478, #951, #2962, #1700, #5226, #4353, #3701, #5033, #3800, #4441, #6667, #4537, #6577, #5834, #7370, #7188, #994, #4492, #2306, #1600, #8626, #5128, #7278, #3752, #904, #210, #2257, #7890, #3060, #1653, #6623, #7324, #5880, #5082, #8717, #2349, #3152, #5179, #250, #8943, #2594, #3334, #439, #8168, #3238, #7420, #8118, #1044, #1937, #6864, #2542, #7609, #6016, #4719, #8811, #4629, #4074, #8213, #488, #7559, #1796, #6062, #7512, #1186, #4030, #4765, #3892, #6164, #1847, #6813, #8898, #8990, #1747, #5274, #5365, #4583, #5412, #6115, #2639, #4675, #6911, #1233, #5460, #535, #3376, #1893, #8305, #1095, #7467, #6763, #2448, #3936, #2493, #6712, #342, #3195, #1141, #8261, #8854, #5315, #390, #3983, #3286, #6951, #2725, #7610, #3239, #6912, #489, #4116, #580, #5366, #536, #3287, #1096, #7655, #8215, #1234, #6210, #7513, #4075, #3377, #2595, #3937, #3424, #8262, #1278, #9039, #8354, #6063, #5413, #8398, #6253 ),
 .UNSPECIFIED., .F., .T. ) 
 B_SPLINE_CURVE_WITH_KNOTS ( ( 3, 2, 2, 2, 2, 2, 2, 2, 2, 2, 2, 2, 2, 2, 2, 2, 2, 2, 2, 2, 2, 2, 2, 2, 2, 2, 2, 2, 2, 2, 2, 2, 2, 2, 2, 2, 2, 2, 2, 2, 2, 2, 2, 2, 2, 2, 2, 2, 2, 2, 2, 2, 2, 2, 2, 2, 2, 2, 2, 2, 2, 2, 2, 2, 2, 2, 2, 2, 2, 2, 2, 2, 3 ),
 ( 0.000000000000000000, 0.01388888888888888812, 0.02777777777777777624, 0.04166666666666666435, 0.05555555555555555247, 0.06944444444444444753, 0.08333333333333332871, 0.09722222222222222376, 0.1111111111111111049, 0.1250000000000000000, 0.1388888888888888951, 0.1527777777777777901, 0.1666666666666666574, 0.1805555555555555525, 0.1944444444444444475, 0.2083333333333333426, 0.2222222222222222099, 0.2361111111111111049, 0.2500000000000000000, 0.2638888888888888951, 0.2777777777777777901, 0.2916666666666666852, 0.3055555555555555802, 0.3194444444444444198, 0.3333333333333333148, 0.3472222222222222099, 0.3611111111111111049, 0.3750000000000000000, 0.3888888888888888951, 0.4027777777777777901, 0.4166666666666666852, 0.4305555555555555802, 0.4444444444444444198, 0.4583333333333333148, 0.4722222222222222099, 0.4861111111111111049, 0.5000000000000000000, 0.5138888888888888395, 0.5277777777777777901, 0.5416666666666666297, 0.5555555555555555802, 0.5694444444444444198, 0.5833333333333333703, 0.5972222222222222099, 0.6111111111111111605, 0.6250000000000000000, 0.6388888888888888395, 0.6527777777777777901, 0.6666666666666666297, 0.6805555555555555802, 0.6944444444444444198, 0.7083333333333333703, 0.7222222222222222099, 0.7361111111111111605, 0.7500000000000000000, 0.7638888888888888395, 0.7777777777777777901, 0.7916666666666666297, 0.8055555555555555802, 0.8194444444444444198, 0.8333333333333333703, 0.8472222222222222099, 0.8611111111111111605, 0.8750000000000000000, 0.8888888888888888395, 0.9027777777777777901, 0.9166666666666666297, 0.9305555555555555802, 0.9444444444444444198, 0.9583333333333333703, 0.9722222222222222099, 0.9861111111111111605, 1.000000000000000000 ),
 .UNSPECIFIED. ) 
 CURVE ( )  GEOMETRIC_REPRESENTATION_ITEM ( )  RATIONAL_B_SPLINE_CURVE ( ( 1.000000000000000000, 0.8660254037844387076, 1.000000000000000000, 0.8660254037844387076, 1.000000000000000000, 0.8660254037844387076, 1.000000000000000000, 0.8660254037844387076, 1.000000000000000000, 0.8660254037844387076, 1.000000000000000000, 0.8660254037844387076, 1.000000000000000000, 0.8660254037844387076, 1.000000000000000000, 0.8660254037844387076, 1.000000000000000000, 0.8660254037844387076, 1.000000000000000000, 0.8660254037844387076, 1.000000000000000000, 0.8660254037844387076, 1.000000000000000000, 0.8660254037844387076, 1.000000000000000000, 0.8660254037844387076, 1.000000000000000000, 0.8660254037844387076, 1.000000000000000000, 0.8660254037844387076, 1.000000000000000000, 0.8660254037844387076, 1.000000000000000000, 0.8660254037844387076, 1.000000000000000000, 0.8660254037844387076, 1.000000000000000000, 0.8660254037844387076, 1.000000000000000000, 0.8660254037844387076, 1.000000000000000000, 0.8660254037844387076, 1.000000000000000000, 0.8660254037844387076, 1.000000000000000000, 0.8660254037844387076, 1.000000000000000000, 0.8660254037844387076, 1.000000000000000000, 0.8660254037844387076, 1.000000000000000000, 0.8660254037844387076, 1.000000000000000000, 0.8660254037844387076, 1.000000000000000000, 0.8660254037844387076, 1.000000000000000000, 0.8660254037844387076, 1.000000000000000000, 0.8660254037844387076, 1.000000000000000000, 0.8660254037844387076, 1.000000000000000000, 0.8660254037844387076, 1.000000000000000000, 0.8660254037844387076, 1.000000000000000000, 0.8660254037844387076, 1.000000000000000000, 0.8660254037844387076, 1.000000000000000000, 0.8660254037844387076, 1.000000000000000000, 0.8660254037844387076, 1.000000000000000000, 0.8660254037844387076, 1.000000000000000000, 0.8660254037844387076, 1.000000000000000000, 0.8660254037844387076, 1.000000000000000000, 0.8660254037844387076, 1.000000000000000000, 0.8660254037844387076, 1.000000000000000000, 0.8660254037844387076, 1.000000000000000000, 0.8660254037844387076, 1.000000000000000000, 0.8660254037844387076, 1.000000000000000000, 0.8660254037844387076, 1.000000000000000000, 0.8660254037844387076, 1.000000000000000000, 0.8660254037844387076, 1.000000000000000000, 0.8660254037844387076, 1.000000000000000000, 0.8660254037844387076, 1.000000000000000000, 0.8660254037844387076, 1.000000000000000000, 0.8660254037844387076, 1.000000000000000000, 0.8660254037844387076, 1.000000000000000000, 0.8660254037844387076, 1.000000000000000000, 0.8660254037844387076, 1.000000000000000000, 0.8660254037844387076, 1.000000000000000000, 0.8660254037844387076, 1.000000000000000000, 0.8660254037844387076, 1.000000000000000000, 0.8660254037844387076, 1.000000000000000000, 0.8660254037844387076, 1.000000000000000000, 0.8660254037844387076, 1.000000000000000000, 0.8660254037844387076, 1.000000000000000000, 0.8660254037844387076, 1.000000000000000000, 0.8660254037844387076, 1.000000000000000000, 0.8660254037844387076, 1.000000000000000000, 0.8660254037844387076, 1.000000000000000000, 0.8660254037844387076, 1.000000000000000000, 0.8660254037844387076, 1.000000000000000000, 0.8660254037844387076, 1.000000000000000000, 0.8660254037844387076, 1.000000000000000000, 0.8660254037844387076, 1.000000000000000000, 0.8660254037844387076, 1.000000000000000000 ) ) 
 REPRESENTATION_ITEM ( '' )  );
#6439=CARTESIAN_POINT ( 'NONE',  ( -5.249999999999999112, -29.02083333333332860, -3.031088913245534755 ) ) ;
#6447=CARTESIAN_POINT ( 'NONE',  ( -3.807688866302469071E-16, -27.42187499965860198, -6.218427825808274356 ) ) ;
#6449=EDGE_CURVE ( 'NONE', #6852, #6768, #6158, .T. ) ;
#6453=CARTESIAN_POINT ( 'NONE',  ( 1.113604000661152470E-15, -29.43750000000000000, 6.062177826491070398 ) ) ;
#6455=CARTESIAN_POINT ( 'NONE',  ( 5.385316468749999252, -27.43229166632526983, -3.109213912904139399 ) ) ;
#6458=EDGE_LOOP ( 'NONE', ( #3236, #1035, #8671, #927, #4684, #6470, #8151, #2254, #2236, #4556, #8403, #3521, #4633, #6219, #3601, #3271, #437, #3650, #4969, #5290, #7396, #8925, #6097, #2648, #6677, #949, #307, #3867 ) ) ;
#6460=DIRECTION ( 'NONE',  ( 0.000000000000000000, 0.000000000000000000, -1.000000000000000000 ) ) ;
#6461=( BOUNDED_CURVE ( )  B_SPLINE_CURVE ( 2, ( #1764, #7437, #7245, #1668, #4511 ),
 .UNSPECIFIED., .F., .F. ) 
 B_SPLINE_CURVE_WITH_KNOTS ( ( 3, 2, 3 ),
 ( 0.000000000000000000, 0.01388888888888888812, 0.02083333333333333218 ),
 .UNSPECIFIED. ) 
 CURVE ( )  GEOMETRIC_REPRESENTATION_ITEM ( )  RATIONAL_B_SPLINE_CURVE ( ( 1.000000000000000000, 0.8660254037844387076, 1.000000000000000000, 0.9330127018922194093, 0.9330127018922194093 ) ) 
 REPRESENTATION_ITEM ( '' )  );
#6470=ORIENTED_EDGE ( 'NONE', *, *, #6337, .F. ) ;
#6471=LINE ( 'NONE', #7971, #7597 ) ;
#6477=CARTESIAN_POINT ( 'NONE',  ( 5.250000000000000888, -29.64583333333333215, 3.031088913245533423 ) ) ;
#6478=CARTESIAN_POINT ( 'NONE',  ( -5.385316468750000141, -27.35937499965860198, 0.000000000000000000 ) ) ;
#6484=( GEOMETRIC_REPRESENTATION_CONTEXT ( 3 ) GLOBAL_UNCERTAINTY_ASSIGNED_CONTEXT ( ( #4405 ) ) GLOBAL_UNIT_ASSIGNED_CONTEXT ( ( #6796, #8248, #4795 ) ) REPRESENTATION_CONTEXT ( 'NONE', 'WORKASPACE' ) );
#6492=CARTESIAN_POINT ( 'NONE',  ( 5.385316468750000141, -27.98437499965860198, -6.595110575850215044E-16 ) ) ;
#6496=ORIENTED_EDGE ( 'NONE', *, *, #2568, .T. ) ;
#6498=CARTESIAN_POINT ( 'NONE',  ( -3.807688866302469071E-16, -27.89062499965860198, -6.218427825808274356 ) ) ;
#6500=CARTESIAN_POINT ( 'NONE',  ( 2.692658234374998738, -27.66145833299193413, -4.663820869356206877 ) ) ;
#6504=CIRCLE ( 'NONE', #7258, 5.250000000000000000 ) ;
#6506=EDGE_CURVE ( 'NONE', #946, #2693, #7702, .T. ) ;
#6524=ORIENTED_EDGE ( 'NONE', *, *, #8673, .T. ) ;
#6526=CARTESIAN_POINT ( 'NONE',  ( -9.180150650966086169E-15, -28.18749999999999645, 5.250000000000000000 ) ) ;
#6531=CARTESIAN_POINT ( 'NONE',  ( 2.624999999999998668, -29.83333333333333215, -4.546633369868303021 ) ) ;
#6533=CARTESIAN_POINT ( 'NONE',  ( -5.385316468750001029, -27.63020833299193413, -3.109213912904136734 ) ) ;
#6537=CARTESIAN_POINT ( 'NONE',  ( 2.692658234375002735, -27.24479166632526628, 4.663820869356205101 ) ) ;
#6543=CARTESIAN_POINT ( 'NONE',  ( -5.250000000000000000, -28.20833333265053255, -3.031088913245534755 ) ) ;
#6546=CARTESIAN_POINT ( 'NONE',  ( 5.249999999999999112, -29.79166666598387181, -3.031088913245536975 ) ) ;
#6547=ORIENTED_EDGE ( 'NONE', *, *, #645, .F. ) ;
#6549=CARTESIAN_POINT ( 'NONE',  ( -2.692658234374996518, -28.28645833299193413, 4.663820869356208654 ) ) ;
#6550=ADVANCED_FACE ( 'NONE', ( #3333, #389 ), #487, .F. ) ;
#6552=CARTESIAN_POINT ( 'NONE',  ( -5.249999999999997335, -28.47916666666666785, 3.031088913245538308 ) ) ;
#6553=VERTEX_POINT ( 'NONE', #5273 ) ;
#6554=CARTESIAN_POINT ( 'NONE',  ( 5.385316468750001029, -27.22395833299193413, 3.109213912904135846 ) ) ;
#6565=CARTESIAN_POINT ( 'NONE',  ( -1.406733260263391960, -27.69866454968462932, 5.250000000000000000 ) ) ;
#6574=AXIS2_PLACEMENT_3D ( 'NONE', #5795, #2927, #4953 ) ;
#6575=( BOUNDED_CURVE ( )  B_SPLINE_CURVE ( 2, ( #5136, #8772, #6531, #857, #3156, #5279, #4543, #3756, #4498 ),
 .UNSPECIFIED., .F., .T. ) 
 B_SPLINE_CURVE_WITH_KNOTS ( ( 3, 2, 2, 2, 3 ),
 ( 0.9375000000000000000, 0.9444444444444444198, 0.9583333333333333703, 0.9722222222222222099, 0.9791666666666667407 ),
 .UNSPECIFIED. ) 
 CURVE ( )  GEOMETRIC_REPRESENTATION_ITEM ( )  RATIONAL_B_SPLINE_CURVE ( ( 0.9330127018922194093, 0.9330127018922194093, 1.000000000000000000, 0.8660254037844387076, 1.000000000000000000, 0.8660254037844387076, 1.000000000000000000, 0.9330127018922187432, 0.9330127018922192983 ) ) 
 REPRESENTATION_ITEM ( '' )  );
#6576=CARTESIAN_POINT ( 'NONE',  ( -1.406733260263394625, -29.80133545031537068, -5.250000000000000000 ) ) ;
#6577=CARTESIAN_POINT ( 'NONE',  ( -5.385316468750000141, -27.60937499965860198, 0.000000000000000000 ) ) ;
#6586=EDGE_CURVE ( 'NONE', #8584, #2823, #1846, .T. ) ;
#6587=CARTESIAN_POINT ( 'NONE',  ( 1.142306659890740623E-15, -27.54687499965860198, 6.218427825808274356 ) ) ;
#6590=CARTESIAN_POINT ( 'NONE',  ( -5.385316468750000141, -27.57812499965860198, 0.000000000000000000 ) ) ;
#6592=CARTESIAN_POINT ( 'NONE',  ( -1.406733260263402174, -29.38616454900182973, 5.249999999999995559 ) ) ;
#6595=CARTESIAN_POINT ( 'NONE',  ( -5.249999999999999112, -27.91666666598387181, 3.031088913245538308 ) ) ;
#6599=CARTESIAN_POINT ( 'NONE',  ( -5.385316468750000141, -27.57812499965860198, 0.000000000000000000 ) ) ;
#6604=CARTESIAN_POINT ( 'NONE',  ( -2.692658234375000514, -27.11979166632526628, -4.663820869356205989 ) ) ;
#6609=CARTESIAN_POINT ( 'NONE',  ( 1.113604000661152470E-15, -27.43750000000000000, 6.062177826491070398 ) ) ;
#6613=CARTESIAN_POINT ( 'NONE',  ( 0.000000000000000000, -50.00000000000000000, 0.000000000000000000 ) ) ;
#6621=LINE ( 'NONE', #249, #3480 ) ;
#6623=CARTESIAN_POINT ( 'NONE',  ( 5.385316468750000141, -27.98437499965860198, -6.595110575850215044E-16 ) ) ;
#6630=CARTESIAN_POINT ( 'NONE',  ( -5.385316468750000141, -27.35937499965860198, 0.000000000000000000 ) ) ;
#6632=ORIENTED_EDGE ( 'NONE', *, *, #4774, .T. ) ;
#6633=CARTESIAN_POINT ( 'NONE',  ( 5.250000000000000000, -28.81249999931720396, -6.429395695523604153E-16 ) ) ;
#6635=CARTESIAN_POINT ( 'NONE',  ( -5.249999999999999112, -27.45833333265053611, -3.031088913245534755 ) ) ;
#6636=CARTESIAN_POINT ( 'NONE',  ( -5.249999999999999112, -27.66666666598386826, 3.031088913245538308 ) ) ;
#6642=CARTESIAN_POINT ( 'NONE',  ( 1.142306659890740623E-15, -28.01562499965860553, 6.218427825808274356 ) ) ;
#6644=CYLINDRICAL_SURFACE ( 'NONE', #2508, 5.250000000000000000 ) ;
#6646=CARTESIAN_POINT ( 'NONE',  ( -2.692658234374996518, -29.03645833299193413, 4.663820869356208654 ) ) ;
#6652=CARTESIAN_POINT ( 'NONE',  ( 5.250000000000000888, -27.64583333333333570, 3.031088913245532979 ) ) ;
#6665=CARTESIAN_POINT ( 'NONE',  ( 1.975475456537005874E-15, -27.93749999999999289, 5.250000000000000000 ) ) ;
#6667=CARTESIAN_POINT ( 'NONE',  ( -2.692658234374996518, -27.56770833299193413, 4.663820869356208654 ) ) ;
#6669=CARTESIAN_POINT ( 'NONE',  ( 5.385316468749999252, -28.46354166632526628, -3.109213912904139399 ) ) ;
#6673=CARTESIAN_POINT ( 'NONE',  ( 1.045839947578414884E-14, -27.99999999931720041, -5.250000000000000000 ) ) ;
#6675=CARTESIAN_POINT ( 'NONE',  ( 2.692658234375002735, -27.77604166632526628, 4.663820869356205101 ) ) ;
#6677=ORIENTED_EDGE ( 'NONE', *, *, #3723, .F. ) ;
#6678=CARTESIAN_POINT ( 'NONE',  ( 1.406733260263403507, -28.76116454900182973, -5.249999999999994671 ) ) ;
#6681=CARTESIAN_POINT ( 'NONE',  ( -5.249999999999999112, -28.41666666598387181, 3.031088913245538308 ) ) ;
#6683=( BOUNDED_CURVE ( )  B_SPLINE_CURVE ( 2, ( #3789, #8614, #3050, #2337, #8662, #5168, #2245, #4480, #5118 ),
 .UNSPECIFIED., .F., .F. ) 
 B_SPLINE_CURVE_WITH_KNOTS ( ( 3, 2, 2, 2, 3 ),
 ( 0.8958333333333333703, 0.9027777777777777901, 0.9166666666666666297, 0.9305555555555555802, 0.9375000002123526910 ),
 .UNSPECIFIED. ) 
 CURVE ( )  GEOMETRIC_REPRESENTATION_ITEM ( )  RATIONAL_B_SPLINE_CURVE ( ( 0.9330127018922192983, 0.9330127018922198534, 1.000000000000000000, 0.8660254037844387076, 1.000000000000000000, 0.8660254037844387076, 1.000000000000000000, 0.9330126998438290631, 0.9330127018922194093 ) ) 
 REPRESENTATION_ITEM ( '' )  );
#6684=CARTESIAN_POINT ( 'NONE',  ( 5.249999999999999112, -29.04166666598387181, -3.031088913245536975 ) ) ;
#6685=DIRECTION ( 'NONE',  ( 1.000000000000000000, 0.000000000000000000, 0.000000000000000000 ) ) ;
#6687=CARTESIAN_POINT ( 'NONE',  ( 5.385316468750001029, -28.47395833299193413, 3.109213912904135846 ) ) ;
#6689=CARTESIAN_POINT ( 'NONE',  ( 6.429395695523604153E-16, -27.00000000000000000, 5.250000000000000000 ) ) ;
#6691=CARTESIAN_POINT ( 'NONE',  ( -5.385316468749998364, -27.80729166632526628, 3.109213912904140287 ) ) ;
#6696=EDGE_CURVE ( 'NONE', #5282, #3224, #6504, .T. ) ;
#6698=VERTEX_POINT ( 'NONE', #4073 ) ;
#6701=EDGE_LOOP ( 'NONE', ( #1580, #8515, #415, #5711 ) ) ;
#6707=EDGE_CURVE ( 'NONE', #8870, #7281, #4248, .T. ) ;
#6712=CARTESIAN_POINT ( 'NONE',  ( 1.142306659890740623E-15, -29.29687499965859487, 6.218427825808274356 ) ) ;
#6714=CARTESIAN_POINT ( 'NONE',  ( 5.385316468750001029, -29.00520833299193413, 3.109213912904135846 ) ) ;
#6718=CARTESIAN_POINT ( 'NONE',  ( 1.142306659890740623E-15, -27.29687499965859843, 6.218427825808274356 ) ) ;
#6722=CARTESIAN_POINT ( 'NONE',  ( 2.692658234375002735, -27.99479166632526628, 4.663820869356205101 ) ) ;
#6728=CARTESIAN_POINT ( 'NONE',  ( 2.624999999999998668, -28.02083333265053255, -4.546633369868303021 ) ) ;
#6734=CARTESIAN_POINT ( 'NONE',  ( -2.692658234374996518, -29.03645833299193413, 4.663820869356208654 ) ) ;
#6737=DIRECTION ( 'NONE',  ( 0.000000000000000000, -1.000000000000000000, 0.000000000000000000 ) ) ;
#6739=CARTESIAN_POINT ( 'NONE',  ( 5.385316468750001029, -27.97395833299193413, 3.109213912904135846 ) ) ;
#6746=( BOUNDED_CURVE ( )  B_SPLINE_CURVE ( 2, ( #3058, #1599, #7226, #4352, #5879, #8716, #3799, #6576, #8625 ),
 .UNSPECIFIED., .F., .F. ) 
 B_SPLINE_CURVE_WITH_KNOTS ( ( 3, 2, 2, 2, 3 ),
 ( 0.8958333333333333703, 0.9027777777777777901, 0.9166666666666666297, 0.9305555555555555802, 0.9375000000000000000 ),
 .UNSPECIFIED. ) 
 CURVE ( )  GEOMETRIC_REPRESENTATION_ITEM ( )  RATIONAL_B_SPLINE_CURVE ( ( 0.9330127018922192983, 0.9330127018922198534, 1.000000000000000000, 0.8660254037844387076, 1.000000000000000000, 0.8660254037844387076, 1.000000000000000000, 0.9330127018922194093, 0.9330127018922194093 ) ) 
 REPRESENTATION_ITEM ( '' )  );
#6750=CARTESIAN_POINT ( 'NONE',  ( 2.624999999999998668, -27.08333333333333570, -4.546633369868303021 ) ) ;
#6751=ADVANCED_FACE ( 'NONE', ( #5550 ), #5509, .F. ) ;
#6756=DIRECTION ( 'NONE',  ( 0.000000000000000000, -1.000000000000000000, 0.000000000000000000 ) ) ;
#6763=CARTESIAN_POINT ( 'NONE',  ( 5.385316468749999252, -29.21354166632527338, -3.109213912904138954 ) ) ;
#6766=CARTESIAN_POINT ( 'NONE',  ( -5.385316468750000141, -29.85937499965859843, 0.000000000000000000 ) ) ;
#6768=VERTEX_POINT ( 'NONE', #6251 ) ;
#6771=EDGE_CURVE ( 'NONE', #8099, #4014, #3375, .T. ) ;
#6772=CARTESIAN_POINT ( 'NONE',  ( 2.692658234374998738, -29.44270833299193413, -4.663820869356206877 ) ) ;
#6773=ORIENTED_EDGE ( 'NONE', *, *, #4774, .F. ) ;
#6774=CARTESIAN_POINT ( 'NONE',  ( -2.692658234374996518, -28.78645833299193413, 4.663820869356208654 ) ) ;
#6784=CARTESIAN_POINT ( 'NONE',  ( 2.692658234375002735, -29.99479166632526628, 4.663820869356205101 ) ) ;
#6786=CARTESIAN_POINT ( 'NONE',  ( -9.180150650966086169E-15, -28.62499999931720396, 5.249999999999999112 ) ) ;
#6787=CARTESIAN_POINT ( 'NONE',  ( -2.692658234374996518, -28.03645833299193413, 4.663820869356208654 ) ) ;
#6789=EDGE_CURVE ( 'NONE', #2434, #8455, #8999, .T. ) ;
#6790=EDGE_LOOP ( 'NONE', ( #7502, #1101 ) ) ;
#6796=( LENGTH_UNIT ( ) NAMED_UNIT ( * ) SI_UNIT ( .MILLI., .METRE. ) );
#6797=CARTESIAN_POINT ( 'NONE',  ( 2.624999999999998668, -27.83333333333333215, -4.546633369868303021 ) ) ;
#6799=EDGE_CURVE ( 'NONE', #6343, #451, #4847, .T. ) ;
#6805=CARTESIAN_POINT ( 'NONE',  ( -5.250000000000000000, -29.18749999931720396, 0.000000000000000000 ) ) ;
#6813=CARTESIAN_POINT ( 'NONE',  ( 1.142306659890740623E-15, -28.79687499965860198, 6.218427825808274356 ) ) ;
#6816=CARTESIAN_POINT ( 'NONE',  ( -2.692658234375000514, -29.65104166632526983, -4.663820869356205989 ) ) ;
#6822=ADVANCED_FACE ( 'NONE', ( #7653 ), #1276, .F. ) ;
#6823=CARTESIAN_POINT ( 'NONE',  ( -5.385316468749998364, -29.08854166632526628, 3.109213912904140287 ) ) ;
#6827=CARTESIAN_POINT ( 'NONE',  ( 2.692658234374998738, -28.91145833299193413, -4.663820869356206877 ) ) ;
#6833=CARTESIAN_POINT ( 'NONE',  ( 2.324088772396477476E-15, -27.31250000000000000, -5.250000000000000000 ) ) ;
#6836=CIRCLE ( 'NONE', #2833, 5.250000000000000000 ) ;
#6838=CARTESIAN_POINT ( 'NONE',  ( -3.807688866302469071E-16, -29.64062499965859843, -6.218427825808274356 ) ) ;
#6841=CARTESIAN_POINT ( 'NONE',  ( -5.385316468749998364, -28.55729166632527338, 3.109213912904140287 ) ) ;
#6844=CARTESIAN_POINT ( 'NONE',  ( 2.625000000000002220, -30.10416666598386826, 4.546633369868302132 ) ) ;
#6845=PRODUCT_DEFINITION_CONTEXT ( 'detailed design', #43, 'design' ) ;
#6850=CARTESIAN_POINT ( 'NONE',  ( 5.250000000000000000, -29.12499999999999645, -6.429395695523604153E-16 ) ) ;
#6852=VERTEX_POINT ( 'NONE', #7252 ) ;
#6857=DIRECTION ( 'NONE',  ( 0.000000000000000000, -1.000000000000000000, 0.000000000000000000 ) ) ;
#6858=ADVANCED_FACE ( 'NONE', ( #7395 ), #6644, .F. ) ;
#6861=DIRECTION ( 'NONE',  ( 1.000000000000000000, 0.000000000000000000, 0.000000000000000000 ) ) ;
#6863=DIRECTION ( 'NONE',  ( 0.000000000000000000, -1.000000000000000000, 0.000000000000000000 ) ) ;
#6864=CARTESIAN_POINT ( 'NONE',  ( -5.385316468750001029, -28.38020833299193413, -3.109213912904136734 ) ) ;
#6867=CARTESIAN_POINT ( 'NONE',  ( 2.692658234375002735, -30.02604166632526983, 4.663820869356205101 ) ) ;
#6873=CARTESIAN_POINT ( 'NONE',  ( -3.807688866302469071E-16, -29.67187499965860198, -6.218427825808274356 ) ) ;
#6875=CARTESIAN_POINT ( 'NONE',  ( 2.692658234375002735, -28.49479166632526628, 4.663820869356205101 ) ) ;
#6878=EDGE_CURVE ( 'NONE', #2431, #8870, #182, .T. ) ;
#6879=CARTESIAN_POINT ( 'NONE',  ( -5.250000000000000000, -28.43749999931720396, 0.000000000000000000 ) ) ;
#6880=CARTESIAN_POINT ( 'NONE',  ( 2.161402558328724325E-14, -28.81250000000000355, -5.250000000000000000 ) ) ;
#6885=CARTESIAN_POINT ( 'NONE',  ( 5.385316468750000141, -29.20312499965859843, -6.595110575850215044E-16 ) ) ;
#6887=CARTESIAN_POINT ( 'NONE',  ( -2.625000000000000444, -29.54166666666666785, -4.546633369868303021 ) ) ;
#6889=CARTESIAN_POINT ( 'NONE',  ( -5.385316468750000141, -29.82812499965859843, 0.000000000000000000 ) ) ;
#6896=EDGE_CURVE ( 'NONE', #7225, #8711, #387, .T. ) ;
#6898=ORIENTED_EDGE ( 'NONE', *, *, #3839, .T. ) ;
#6899=( NAMED_UNIT ( * ) SI_UNIT ( $, .STERADIAN. ) SOLID_ANGLE_UNIT ( ) );
#6900=CARTESIAN_POINT ( 'NONE',  ( 1.113604000661152470E-15, -28.43750000000000355, 6.062177826491070398 ) ) ;
#6906=CARTESIAN_POINT ( 'NONE',  ( -2.624999999999996891, -29.95833333333333215, 4.546633369868304797 ) ) ;
#6910=CARTESIAN_POINT ( 'NONE',  ( -2.625000000000000444, -29.29166666666666785, -4.546633369868303021 ) ) ;
#6911=CARTESIAN_POINT ( 'NONE',  ( 2.692658234375002735, -29.02604166632526983, 4.663820869356205101 ) ) ;
#6912=CARTESIAN_POINT ( 'NONE',  ( -5.385316468749998364, -29.58854166632527694, 3.109213912904140287 ) ) ;
#6914=CARTESIAN_POINT ( 'NONE',  ( -2.692658234374996518, -28.81770833299193413, 4.663820869356208654 ) ) ;
#6917=EDGE_LOOP ( 'NONE', ( #4587, #7804, #7045, #3820 ) ) ;
#6918=CARTESIAN_POINT ( 'NONE',  ( 2.324088772396477476E-15, -27.31250000000000000, -5.250000000000000000 ) ) ;
#6920=CARTESIAN_POINT ( 'NONE',  ( -5.385316468749998364, -28.83854166632526628, 3.109213912904140287 ) ) ;
#6922=CARTESIAN_POINT ( 'NONE',  ( -5.385316468750000141, -28.57812499965860198, 0.000000000000000000 ) ) ;
#6930=CARTESIAN_POINT ( 'NONE',  ( 1.142306659890740623E-15, -29.01562499965860198, 6.218427825808274356 ) ) ;
#6932=DIRECTION ( 'NONE',  ( 0.000000000000000000, -1.000000000000000000, 0.000000000000000000 ) ) ;
#6933=CARTESIAN_POINT ( 'NONE',  ( -3.807688866302469071E-16, -29.64062499965859843, -6.218427825808274356 ) ) ;
#6935=DIRECTION ( 'NONE',  ( 0.000000000000000000, -1.000000000000000000, 0.000000000000000000 ) ) ;
#6938=CARTESIAN_POINT ( 'NONE',  ( -2.625000000000000444, -28.54166666666666785, -4.546633369868303021 ) ) ;
#6941=LINE ( 'NONE', #3414, #4355 ) ;
#6949=CARTESIAN_POINT ( 'NONE',  ( 2.161402558328724325E-14, -29.31250000000000000, -5.250000000000000000 ) ) ;
#6950=CARTESIAN_POINT ( 'NONE',  ( 5.250000000000000888, -28.58333333265053611, 3.031088913245532979 ) ) ;
#6951=CARTESIAN_POINT ( 'NONE',  ( 5.385316468750001029, -29.50520833299193413, 3.109213912904134958 ) ) ;
#6956=CARTESIAN_POINT ( 'NONE',  ( 1.045839947578414884E-14, -27.99999999931720041, -5.249999999999999112 ) ) ;
#6958=CARTESIAN_POINT ( 'NONE',  ( -5.385316468750001029, -28.88020833299193768, -3.109213912904136734 ) ) ;
#6961=CARTESIAN_POINT ( 'NONE',  ( 5.385316468750000141, -29.20312499965859843, -6.595110575850215044E-16 ) ) ;
#6964=VECTOR ( 'NONE', #1674, 1000.000000000000000 ) ;
#6965=ADVANCED_FACE ( 'NONE', ( #7445 ), #8696, .F. ) ;
#6966=ADVANCED_FACE ( 'NONE', ( #1626 ), #7303, .F. ) ;
#6971=CARTESIAN_POINT ( 'NONE',  ( -2.625000000000000444, -28.22916666598386826, -4.546633369868303021 ) ) ;
#6972=CARTESIAN_POINT ( 'NONE',  ( -1.406733260263384411, -28.73883544963257464, -5.250000000000006217 ) ) ;
#6974=CARTESIAN_POINT ( 'NONE',  ( -6.150365299726402968E-16, -50.00000000000000000, 3.794308781941904574 ) ) ;
#6975=CARTESIAN_POINT ( 'NONE',  ( -2.692658234375000514, -29.86979166632526983, -4.663820869356205989 ) ) ;
#6984=CARTESIAN_POINT ( 'NONE',  ( 2.625000000000002220, -28.91666666666666785, 4.546633369868302132 ) ) ;
#6994=SHAPE_REPRESENTATION ( 'cone', ( #888 ), #6484 ) ;
#6995=CARTESIAN_POINT ( 'NONE',  ( 2.625000000000002220, -28.60416666598386826, 4.546633369868302132 ) ) ;
#7005=CARTESIAN_POINT ( 'NONE',  ( -5.385316468749998364, -30.08854166632526983, 3.109213912904140287 ) ) ;
#7007=CARTESIAN_POINT ( 'NONE',  ( -2.692658234374996518, -30.03645833299193413, 4.663820869356208654 ) ) ;
#7014=CARTESIAN_POINT ( 'NONE',  ( -1.406733260263391960, -28.13616454900183328, 5.250000000000000000 ) ) ;
#7015=CARTESIAN_POINT ( 'NONE',  ( 1.975475456537005874E-15, -27.87499999931720041, 5.250000000000000000 ) ) ;
#7018=CARTESIAN_POINT ( 'NONE',  ( 1.975475456537005874E-15, -28.68749999999999645, 5.250000000000000000 ) ) ;
#7019=CARTESIAN_POINT ( 'NONE',  ( -5.385316468749998364, -29.80729166632526628, 3.109213912904140287 ) ) ;
#7022=AXIS2_PLACEMENT_3D ( 'NONE', #334, #7601, #2532 ) ;
#7026=CARTESIAN_POINT ( 'NONE',  ( -2.624999999999996891, -29.45833333333333215, 4.546633369868304797 ) ) ;
#7027=EDGE_CURVE ( 'NONE', #2212, #7281, #3819, .T. ) ;
#7035=CIRCLE ( 'NONE', #8670, 5.242490174541154069 ) ;
#7039=CARTESIAN_POINT ( 'NONE',  ( -2.625000000000000444, -29.47916666598386826, -4.546633369868303021 ) ) ;
#7045=ORIENTED_EDGE ( 'NONE', *, *, #1617, .T. ) ;
#7048=( BOUNDED_CURVE ( )  B_SPLINE_CURVE ( 2, ( #4461, #5200, #7343, #6546, #8644, #2275, #4417, #1670, #967 ),
 .UNSPECIFIED., .F., .F. ) 
 B_SPLINE_CURVE_WITH_KNOTS ( ( 3, 2, 2, 2, 3 ),
 ( 0.8541666666666667407, 0.8611111111111111605, 0.8750000000000000000, 0.8888888888888888395, 0.8958333333333333703 ),
 .UNSPECIFIED. ) 
 CURVE ( )  GEOMETRIC_REPRESENTATION_ITEM ( )  RATIONAL_B_SPLINE_CURVE ( ( 0.9330127018922192983, 0.9330127018922198534, 1.000000000000000000, 0.8660254037844387076, 1.000000000000000000, 0.8660254037844387076, 1.000000000000000000, 0.9330127018922187432, 0.9330127018922192983 ) ) 
 REPRESENTATION_ITEM ( '' )  );
#7049=ORIENTED_EDGE ( 'NONE', *, *, #3015, .T. ) ;
#7050=FACE_OUTER_BOUND ( 'NONE', #1923, .T. ) ;
#7056=CARTESIAN_POINT ( 'NONE',  ( 2.624999999999998668, -27.27083333265053611, -4.546633369868303021 ) ) ;
#7058=CARTESIAN_POINT ( 'NONE',  ( 1.406733260263398400, -28.26116454900183328, -5.249999999999997335 ) ) ;
#7062=DIRECTION ( 'NONE',  ( 0.000000000000000000, 0.000000000000000000, -1.000000000000000000 ) ) ;
#7063=CARTESIAN_POINT ( 'NONE',  ( -2.692658234374996518, -29.28645833299193413, 4.663820869356208654 ) ) ;
#7069=CARTESIAN_POINT ( 'NONE',  ( -5.249999999999999112, -29.72916666666667140, 3.031088913245538308 ) ) ;
#7070=ADVANCED_FACE ( 'NONE', ( #2662 ), #3404, .F. ) ;
#7075=CARTESIAN_POINT ( 'NONE',  ( 0.000000000000000000, -27.00000000000000000, 0.000000000000000000 ) ) ;
#7076=EDGE_CURVE ( 'NONE', #2627, #7114, #1952, .T. ) ;
#7080=DIRECTION ( 'NONE',  ( 0.000000000000000000, -1.000000000000000000, 0.000000000000000000 ) ) ;
#7081=CARTESIAN_POINT ( 'NONE',  ( -3.712013335537174572E-16, -29.74999999931720041, -6.062177826491070398 ) ) ;
#7082=DIRECTION ( 'NONE',  ( 0.000000000000000000, 0.000000000000000000, -1.000000000000000000 ) ) ;
#7091=VERTEX_POINT ( 'NONE', #6974 ) ;
#7092=CARTESIAN_POINT ( 'NONE',  ( 1.142306659890740623E-15, -29.26562499965859843, 6.218427825808274356 ) ) ;
#7098=DIRECTION ( 'NONE',  ( 0.000000000000000000, -1.000000000000000000, 0.000000000000000000 ) ) ;
#7102=CYLINDRICAL_SURFACE ( 'NONE', #1093, 5.250000000000000000 ) ;
#7107=CARTESIAN_POINT ( 'NONE',  ( -2.692658234374996518, -27.56770833299193413, 4.663820869356208654 ) ) ;
#7113=CARTESIAN_POINT ( 'NONE',  ( -3.807688866302469071E-16, -27.39062499965860198, -6.218427825808274356 ) ) ;
#7114=VERTEX_POINT ( 'NONE', #6786 ) ;
#7116=CARTESIAN_POINT ( 'NONE',  ( -5.385316468750001029, -27.09895833299193413, -3.109213912904136734 ) ) ;
#7120=CARTESIAN_POINT ( 'NONE',  ( 0.000000000000000000, -27.00000000000000000, 0.000000000000000000 ) ) ;
#7121=( BOUNDED_CURVE ( )  B_SPLINE_CURVE ( 2, ( #7923, #8060, #842, #2246, #942, #8708, #3644, #985, #2294 ),
 .UNSPECIFIED., .F., .T. ) 
 B_SPLINE_CURVE_WITH_KNOTS ( ( 3, 2, 2, 2, 3 ),
 ( 0.3958333333333333703, 0.4027777777777777901, 0.4166666666666666852, 0.4305555555555555802, 0.4375000000000000000 ),
 .UNSPECIFIED. ) 
 CURVE ( )  GEOMETRIC_REPRESENTATION_ITEM ( )  RATIONAL_B_SPLINE_CURVE ( ( 0.9330127018922194093, 0.9330127018922196314, 1.000000000000000000, 0.8660254037844387076, 1.000000000000000000, 0.8660254037844387076, 1.000000000000000000, 0.9330127018922194093, 0.9330127018922194093 ) ) 
 REPRESENTATION_ITEM ( '' )  );
#7124=CLOSED_SHELL ( 'NONE', ( #206, #5426, #8362, #6822, #971, #6238, #194, #4133, #481, #6751, #5483, #6965, #7486, #8941, #1867, #1436, #3692, #486, #7675, #6858, #7704, #713, #7070, #1169, #3621, #4957, #5164, #7358, #4343, #5618, #6550, #3850, #8677, #8212, #5374, #6966, #4659, #4190, #5878, #3886 ) ) ;
#7127=CARTESIAN_POINT ( 'NONE',  ( 1.113604000661152470E-15, -29.12499999931720751, 6.062177826491070398 ) ) ;
#7128=CARTESIAN_POINT ( 'NONE',  ( 2.624999999999998668, -27.52083333265053611, -4.546633369868303021 ) ) ;
#7136=CARTESIAN_POINT ( 'NONE',  ( 5.249999999999999112, -28.04166666598386826, -3.031088913245536975 ) ) ;
#7141=ORIENTED_EDGE ( 'NONE', *, *, #2253, .T. ) ;
#7142=CARTESIAN_POINT ( 'NONE',  ( 1.142306659890740623E-15, -30.01562499965859843, 6.218427825808274356 ) ) ;
#7144=CARTESIAN_POINT ( 'NONE',  ( 1.975475456537005874E-15, -27.62499999931720041, 5.249999999999999112 ) ) ;
#7147=CARTESIAN_POINT ( 'NONE',  ( 0.000000000000000000, -30.00000000000000000, 0.000000000000000000 ) ) ;
#7148=CARTESIAN_POINT ( 'NONE',  ( 5.385316468750001029, -27.25520833299193413, 3.109213912904135846 ) ) ;
#7150=EDGE_CURVE ( 'NONE', #2693, #4496, #982, .T. ) ;
#7152=CARTESIAN_POINT ( 'NONE',  ( 1.406733260263395735, -27.86383544963257464, 5.250000000000000000 ) ) ;
#7155=CARTESIAN_POINT ( 'NONE',  ( 2.692658234375002735, -28.02604166632526628, 4.663820869356205101 ) ) ;
#7159=VERTEX_POINT ( 'NONE', #8190 ) ;
#7160=CARTESIAN_POINT ( 'NONE',  ( 5.385316468749999252, -27.43229166632526983, -3.109213912904139399 ) ) ;
#7162=CARTESIAN_POINT ( 'NONE',  ( 1.975475456537005874E-15, -27.18750000000000000, 5.250000000000000000 ) ) ;
#7167=EDGE_CURVE ( 'NONE', #7319, #6852, #4199, .T. ) ;
#7172=CARTESIAN_POINT ( 'NONE',  ( 1.113604000661152470E-15, -30.12499999931720041, 6.062177826491070398 ) ) ;
#7188=CARTESIAN_POINT ( 'NONE',  ( -3.807688866302469071E-16, -27.67187499965860198, -6.218427825808274356 ) ) ;
#7191=ORIENTED_EDGE ( 'NONE', *, *, #2445, .T. ) ;
#7199=CYLINDRICAL_SURFACE ( 'NONE', #3112, 5.250000000000000000 ) ;
#7200=CARTESIAN_POINT ( 'NONE',  ( 5.385316468750001029, -28.00520833299193413, 3.109213912904135846 ) ) ;
#7204=CARTESIAN_POINT ( 'NONE',  ( 1.406733260263403507, -29.01116454900182973, -5.249999999999994671 ) ) ;
#7205=EDGE_LOOP ( 'NONE', ( #8715, #3181, #764, #4257 ) ) ;
#7206=CARTESIAN_POINT ( 'NONE',  ( 2.692658234374998738, -27.16145833299193413, -4.663820869356206877 ) ) ;
#7208=CARTESIAN_POINT ( 'NONE',  ( -5.385316468749998364, -27.55729166632526628, 3.109213912904140287 ) ) ;
#7212=CARTESIAN_POINT ( 'NONE',  ( 1.406733260263395735, -29.42633545031537423, 5.250000000000000000 ) ) ;
#7225=VERTEX_POINT ( 'NONE', #6223 ) ;
#7226=CARTESIAN_POINT ( 'NONE',  ( -2.624999999999996891, -29.70833333333333215, 4.546633369868304797 ) ) ;
#7227=CARTESIAN_POINT ( 'NONE',  ( -2.692658234375000514, -27.15104166632526628, -4.663820869356205989 ) ) ;
#7230=ORIENTED_EDGE ( 'NONE', *, *, #1645, .T. ) ;
#7235=CARTESIAN_POINT ( 'NONE',  ( -3.807688866302469071E-16, -27.42187499965860198, -6.218427825808274356 ) ) ;
#7244=CARTESIAN_POINT ( 'NONE',  ( -3.712013335537174572E-16, -27.49999999931720041, -6.062177826491070398 ) ) ;
#7245=CARTESIAN_POINT ( 'NONE',  ( -2.625000000000000444, -27.04166666666666430, -4.546633369868303021 ) ) ;
#7250=CARTESIAN_POINT ( 'NONE',  ( 5.385316468749999252, -27.68229166632526272, -3.109213912904139399 ) ) ;
#7252=CARTESIAN_POINT ( 'NONE',  ( 2.161402558328724325E-14, -29.56250000000000355, -5.250000000000000000 ) ) ;
#7254=CARTESIAN_POINT ( 'NONE',  ( 0.000000000000000000, -27.00000000000000000, 0.000000000000000000 ) ) ;
#7258=AXIS2_PLACEMENT_3D ( 'NONE', #3151, #6863, #5969 ) ;
#7262=CARTESIAN_POINT ( 'NONE',  ( -5.249999999999999112, -27.72916666666666785, 3.031088913245538308 ) ) ;
#7263=CARTESIAN_POINT ( 'NONE',  ( -5.250000000000000000, -29.95833333265053611, -3.031088913245534755 ) ) ;
#7266=DIRECTION ( 'NONE',  ( -0.000000000000000000, -1.000000000000000000, -0.000000000000000000 ) ) ;
#7269=EDGE_CURVE ( 'NONE', #8711, #2434, #5134, .T. ) ;
#7271=CARTESIAN_POINT ( 'NONE',  ( 2.625000000000002220, -28.10416666598386826, 4.546633369868302132 ) ) ;
#7277=LINE ( 'NONE', #1652, #1105 ) ;
#7278=CARTESIAN_POINT ( 'NONE',  ( -2.692658234374996518, -27.81770833299193413, 4.663820869356208654 ) ) ;
#7281=VERTEX_POINT ( 'NONE', #1429 ) ;
#7283=CARTESIAN_POINT ( 'NONE',  ( -5.250000000000000000, -27.93749999931720396, 0.000000000000000000 ) ) ;
#7285=CARTESIAN_POINT ( 'NONE',  ( -3.807688866302469071E-16, -27.92187499965860198, -6.218427825808274356 ) ) ;
#7289=CARTESIAN_POINT ( 'NONE',  ( 1.142306659890740623E-15, -27.51562499965860198, 6.218427825808274356 ) ) ;
#7294=CARTESIAN_POINT ( 'NONE',  ( -5.250000000000000000, -27.68749999931720396, 0.000000000000000000 ) ) ;
#7301=CARTESIAN_POINT ( 'NONE',  ( -2.692658234375000514, -28.61979166632526628, -4.663820869356205989 ) ) ;
#7303=PLANE ( 'NONE',  #7406 ) ;
#7312=CARTESIAN_POINT ( 'NONE',  ( -2.624999999999996891, -27.20833333333333570, 4.546633369868304797 ) ) ;
#7316=CARTESIAN_POINT ( 'NONE',  ( -1.406733260263389518, -27.80133545031536357, -5.250000000000001776 ) ) ;
#7319=VERTEX_POINT ( 'NONE', #3532 ) ;
#7324=CARTESIAN_POINT ( 'NONE',  ( 5.385316468750001029, -28.00520833299193768, 3.109213912904134958 ) ) ;
#7327=CARTESIAN_POINT ( 'NONE',  ( 5.250000000000000000, -29.31249999931720041, -6.429395695523604153E-16 ) ) ;
#7330=VECTOR ( 'NONE', #6350, 1000.000000000000000 ) ;
#7332=CARTESIAN_POINT ( 'NONE',  ( -2.692658234374996518, -27.81770833299193413, 4.663820869356208654 ) ) ;
#7335=CARTESIAN_POINT ( 'NONE',  ( -5.385316468750000141, -27.32812499965860198, 0.000000000000000000 ) ) ;
#7339=CARTESIAN_POINT ( 'NONE',  ( 5.250000000000000000, -28.06249999931720396, -6.429395695523604153E-16 ) ) ;
#7342=( BOUNDED_CURVE ( )  B_SPLINE_CURVE ( 2, ( #4340, #6565, #2438, #8757, #800, #7967, #5070, #7316, #7878 ),
 .UNSPECIFIED., .F., .T. ) 
 B_SPLINE_CURVE_WITH_KNOTS ( ( 3, 2, 2, 2, 3 ),
 ( 0.2291666666666666574, 0.2361111111111111049, 0.2500000000000000000, 0.2638888888888888951, 0.2708333333333333703 ),
 .UNSPECIFIED. ) 
 CURVE ( )  GEOMETRIC_REPRESENTATION_ITEM ( )  RATIONAL_B_SPLINE_CURVE ( ( 0.9330127018922194093, 0.9330127018922194093, 1.000000000000000000, 0.8660254037844387076, 1.000000000000000000, 0.8660254037844387076, 1.000000000000000000, 0.9330127018922190762, 0.9330127018922194093 ) ) 
 REPRESENTATION_ITEM ( '' )  );
#7343=CARTESIAN_POINT ( 'NONE',  ( 2.624999999999998668, -29.77083333265053611, -4.546633369868303021 ) ) ;
#7345=CARTESIAN_POINT ( 'NONE',  ( -5.385316468750000141, -28.07812499965860198, 0.000000000000000000 ) ) ;
#7348=VERTEX_POINT ( 'NONE', #5616 ) ;
#7349=CARTESIAN_POINT ( 'NONE',  ( -3.807688866302469071E-16, -28.14062499965860198, -6.218427825808274356 ) ) ;
#7356=CARTESIAN_POINT ( 'NONE',  ( -5.250000000000000000, -27.75000000000000000, 0.000000000000000000 ) ) ;
#7357=CARTESIAN_POINT ( 'NONE',  ( -5.250000000000000000, -30.18749999931720041, 0.000000000000000000 ) ) ;
#7358=ADVANCED_FACE ( 'NONE', ( #8509 ), #7199, .F. ) ;
#7360=DIRECTION ( 'NONE',  ( 0.000000000000000000, -0.000000000000000000, -1.000000000000000000 ) ) ;
#7370=CARTESIAN_POINT ( 'NONE',  ( -2.692658234375000514, -27.65104166632526628, -4.663820869356205989 ) ) ;
#7372=CARTESIAN_POINT ( 'NONE',  ( 1.406733260263393293, -29.26116454900183328, -5.250000000000000000 ) ) ;
#7373=CARTESIAN_POINT ( 'NONE',  ( 2.692658234374998738, -28.19270833299193413, -4.663820869356206877 ) ) ;
#7377=CARTESIAN_POINT ( 'NONE',  ( -5.385316468750001029, -28.13020833299193058, -3.109213912904136734 ) ) ;
#7379=VERTEX_POINT ( 'NONE', #4997 ) ;
#7385=EDGE_CURVE ( 'NONE', #301, #8385, #5733, .T. ) ;
#7386=CARTESIAN_POINT ( 'NONE',  ( -5.250000000000000000, -27.93749999931720396, 0.000000000000000000 ) ) ;
#7389=CARTESIAN_POINT ( 'NONE',  ( 5.250000000000000888, -29.08333333265053611, 3.031088913245533423 ) ) ;
#7393=CARTESIAN_POINT ( 'NONE',  ( -2.692658234374996518, -28.53645833299193413, 4.663820869356208654 ) ) ;
#7395=FACE_OUTER_BOUND ( 'NONE', #3612, .T. ) ;
#7396=ORIENTED_EDGE ( 'NONE', *, *, #6506, .F. ) ;
#7397=CARTESIAN_POINT ( 'NONE',  ( 5.385316468749999252, -28.18229166632526628, -3.109213912904139399 ) ) ;
#7399=ORIENTED_EDGE ( 'NONE', *, *, #9001, .F. ) ;
#7401=( BOUNDED_CURVE ( )  B_SPLINE_CURVE ( 2, ( #7643, #5499, #4109, #8346, #570, #1557, #7975, #1509, #6526 ),
 .UNSPECIFIED., .F., .T. ) 
 B_SPLINE_CURVE_WITH_KNOTS ( ( 3, 2, 2, 2, 3 ),
 ( 0.3541666666666666852, 0.3611111111111111049, 0.3750000000000000000, 0.3888888888888888951, 0.3958333333333333703 ),
 .UNSPECIFIED. ) 
 CURVE ( )  GEOMETRIC_REPRESENTATION_ITEM ( )  RATIONAL_B_SPLINE_CURVE ( ( 0.9330127018922194093, 0.9330127018922196314, 1.000000000000000000, 0.8660254037844387076, 1.000000000000000000, 0.8660254037844387076, 1.000000000000000000, 0.9330127018922190762, 0.9330127018922194093 ) ) 
 REPRESENTATION_ITEM ( '' )  );
#7404=CARTESIAN_POINT ( 'NONE',  ( -5.250000000000000000, -27.27083333333333215, -3.031088913245534755 ) ) ;
#7405=ORIENTED_EDGE ( 'NONE', *, *, #144, .T. ) ;
#7406=AXIS2_PLACEMENT_3D ( 'NONE', #368, #1579, #231 ) ;
#7410=CARTESIAN_POINT ( 'NONE',  ( 0.000000000000000000, -27.00000000000000000, -5.250000000000000000 ) ) ;
#7413=EDGE_LOOP ( 'NONE', ( #2034, #4896, #2163, #7839 ) ) ;
#7417=ORIENTED_EDGE ( 'NONE', *, *, #1329, .F. ) ;
#7420=CARTESIAN_POINT ( 'NONE',  ( 1.142306659890740623E-15, -28.29687499965860553, 6.218427825808274356 ) ) ;
#7424=CARTESIAN_POINT ( 'NONE',  ( 5.385316468750000141, -28.23437499965860198, -6.595110575850215044E-16 ) ) ;
#7426=CARTESIAN_POINT ( 'NONE',  ( 2.625000000000002220, -28.41666666666666785, 4.546633369868302132 ) ) ;
#7428=CARTESIAN_POINT ( 'NONE',  ( 1.142306659890740623E-15, -28.54687499965860198, 6.218427825808274356 ) ) ;
#7432=CARTESIAN_POINT ( 'NONE',  ( -5.385316468749998364, -28.80729166632526272, 3.109213912904140287 ) ) ;
#7436=CARTESIAN_POINT ( 'NONE',  ( -3.712013335537174572E-16, -27.24999999931720041, -6.062177826491070398 ) ) ;
#7437=CARTESIAN_POINT ( 'NONE',  ( -5.249999999999999112, -27.02083333333334281, -3.031088913245534755 ) ) ;
#7443=CARTESIAN_POINT ( 'NONE',  ( -5.385316468749998364, -28.30729166632526628, 3.109213912904140287 ) ) ;
#7445=FACE_OUTER_BOUND ( 'NONE', #71, .T. ) ;
#7447=CARTESIAN_POINT ( 'NONE',  ( -5.385316468750000141, -28.07812499965860198, 0.000000000000000000 ) ) ;
#7455=CARTESIAN_POINT ( 'NONE',  ( -5.250000000000000000, -27.02083333333333570, -3.031088913245534755 ) ) ;
#7461=DIRECTION ( 'NONE',  ( 0.000000000000000000, -1.000000000000000000, 0.000000000000000000 ) ) ;
#7467=CARTESIAN_POINT ( 'NONE',  ( 2.692658234374998738, -29.19270833299193413, -4.663820869356206877 ) ) ;
#7468=CIRCLE ( 'NONE', #5086, 5.250000000000000000 ) ;
#7470=CARTESIAN_POINT ( 'NONE',  ( 5.385316468750000141, -29.48437499965859843, -6.595110575850215044E-16 ) ) ;
#7474=CARTESIAN_POINT ( 'NONE',  ( -2.692658234374996518, -29.31770833299193413, 4.663820869356208654 ) ) ;
#7477=CARTESIAN_POINT ( 'NONE',  ( -3.807688866302469071E-16, -27.89062499965860198, -6.218427825808274356 ) ) ;
#7481=( BOUNDED_CURVE ( )  B_SPLINE_CURVE ( 2, ( #4634, #4772, #6021, #8950, #3342, #9045, #7426, #5418, #8858 ),
 .UNSPECIFIED., .F., .T. ) 
 B_SPLINE_CURVE_WITH_KNOTS ( ( 3, 2, 2, 2, 3 ),
 ( 0.4375000000000000000, 0.4444444444444444198, 0.4583333333333333148, 0.4722222222222222099, 0.4791666666666666852 ),
 .UNSPECIFIED. ) 
 CURVE ( )  GEOMETRIC_REPRESENTATION_ITEM ( )  RATIONAL_B_SPLINE_CURVE ( ( 0.9330127018922194093, 0.9330127018922194093, 1.000000000000000000, 0.8660254037844387076, 1.000000000000000000, 0.8660254037844387076, 1.000000000000000000, 0.9330127018922190762, 0.9330127018922194093 ) ) 
 REPRESENTATION_ITEM ( '' )  );
#7486=ADVANCED_FACE ( 'NONE', ( #4550 ), #3857, .F. ) ;
#7490=CARTESIAN_POINT ( 'NONE',  ( 5.385316468749999252, -29.93229166632526983, -3.109213912904139399 ) ) ;
#7494=CARTESIAN_POINT ( 'NONE',  ( -3.807688866302469071E-16, -28.39062499965859843, -6.218427825808274356 ) ) ;
#7501=CARTESIAN_POINT ( 'NONE',  ( -5.250000000000000000, -28.27083333333332860, -3.031088913245534755 ) ) ;
#7502=ORIENTED_EDGE ( 'NONE', *, *, #435, .F. ) ;
#7510=ORIENTED_EDGE ( 'NONE', *, *, #2944, .T. ) ;
#7512=CARTESIAN_POINT ( 'NONE',  ( -2.692658234375000514, -28.65104166632526628, -4.663820869356205989 ) ) ;
#7513=CARTESIAN_POINT ( 'NONE',  ( -5.385316468749998364, -29.83854166632526983, 3.109213912904140287 ) ) ;
#7515=CARTESIAN_POINT ( 'NONE',  ( 5.385316468750000141, -28.73437499965860198, -6.595110575850215044E-16 ) ) ;
#7518=CARTESIAN_POINT ( 'NONE',  ( 1.975475456537005874E-15, -27.43750000000000000, 5.250000000000000000 ) ) ;
#7520=CARTESIAN_POINT ( 'NONE',  ( -5.385316468749998364, -29.33854166632526983, 3.109213912904140287 ) ) ;
#7522=CARTESIAN_POINT ( 'NONE',  ( -2.692658234375000514, -28.86979166632526983, -4.663820869356205989 ) ) ;
#7528=DIRECTION ( 'NONE',  ( 0.000000000000000000, -1.000000000000000000, 0.000000000000000000 ) ) ;
#7532=CARTESIAN_POINT ( 'NONE',  ( -5.385316468750000141, -29.32812499965859843, 0.000000000000000000 ) ) ;
#7536=( BOUNDED_CURVE ( )  B_SPLINE_CURVE ( 2, ( #3706, #8124, #7940, #3107, #7283, #5088, #164, #3656, #6673 ),
 .UNSPECIFIED., .F., .T. ) 
 B_SPLINE_CURVE_WITH_KNOTS ( ( 3, 2, 2, 2, 3 ),
 ( 0.2291666666666666574, 0.2361111111111111049, 0.2500000000000000000, 0.2638888888888888951, 0.2708333333333333703 ),
 .UNSPECIFIED. ) 
 CURVE ( )  GEOMETRIC_REPRESENTATION_ITEM ( )  RATIONAL_B_SPLINE_CURVE ( ( 0.9330127018922194093, 0.9330127018922194093, 1.000000000000000000, 0.8660254037844387076, 1.000000000000000000, 0.8660254037844387076, 1.000000000000000000, 0.9330127018922190762, 0.9330127018922194093 ) ) 
 REPRESENTATION_ITEM ( '' )  );
#7537=CARTESIAN_POINT ( 'NONE',  ( 5.385316468750000141, -28.95312499965860198, -6.595110575850215044E-16 ) ) ;
#7542=CARTESIAN_POINT ( 'NONE',  ( -5.250000000000000000, -30.18749999931720041, 0.000000000000000000 ) ) ;
#7545=SURFACE_STYLE_USAGE ( .BOTH. , #2762 ) ;
#7546=CARTESIAN_POINT ( 'NONE',  ( 2.624999999999998668, -29.08333333333333215, -4.546633369868303021 ) ) ;
#7559=CARTESIAN_POINT ( 'NONE',  ( -5.385316468749998364, -28.58854166632526628, 3.109213912904140287 ) ) ;
#7563=CARTESIAN_POINT ( 'NONE',  ( -2.692658234374996518, -29.31770833299193413, 4.663820869356208654 ) ) ;
#7567=CARTESIAN_POINT ( 'NONE',  ( -2.624999999999996891, -27.45833333333333570, 4.546633369868304797 ) ) ;
#7569=CARTESIAN_POINT ( 'NONE',  ( 5.385316468750000141, -28.73437499965860198, -6.595110575850215044E-16 ) ) ;
#7570=VERTEX_POINT ( 'NONE', #310 ) ;
#7571=AXIS2_PLACEMENT_3D ( 'NONE', #4089, #6222, #1995 ) ;
#7572=CARTESIAN_POINT ( 'NONE',  ( 5.385316468749999252, -28.43229166632526272, -3.109213912904138954 ) ) ;
#7574=DIRECTION ( 'NONE',  ( 0.000000000000000000, -1.000000000000000000, 0.000000000000000000 ) ) ;
#7582=CARTESIAN_POINT ( 'NONE',  ( 1.975475456537005874E-15, -27.37499999931720041, 5.249999999999999112 ) ) ;
#7585=CARTESIAN_POINT ( 'NONE',  ( -5.385316468750000141, -30.07812499965859843, 0.000000000000000000 ) ) ;
#7587=CARTESIAN_POINT ( 'NONE',  ( -5.249999999999997335, -27.97916666666666430, 3.031088913245538308 ) ) ;
#7588=CARTESIAN_POINT ( 'NONE',  ( 5.385316468750000141, -29.45312499965859843, -6.595110575850215044E-16 ) ) ;
#7596=CARTESIAN_POINT ( 'NONE',  ( 2.624999999999998668, -28.83333333333333215, -4.546633369868303021 ) ) ;
#7597=VECTOR ( 'NONE', #2250, 1000.000000000000000 ) ;
#7598=ORIENTED_EDGE ( 'NONE', *, *, #6449, .T. ) ;
#7601=DIRECTION ( 'NONE',  ( 0.000000000000000000, 0.000000000000000000, -1.000000000000000000 ) ) ;
#7608=CARTESIAN_POINT ( 'NONE',  ( 1.045839947578414884E-14, -27.81249999999999289, -5.250000000000000000 ) ) ;
#7609=CARTESIAN_POINT ( 'NONE',  ( -3.807688866302469071E-16, -28.42187499965860198, -6.218427825808274356 ) ) ;
#7610=CARTESIAN_POINT ( 'NONE',  ( 1.142306659890740623E-15, -29.54687499965859487, 6.218427825808274356 ) ) ;
#7612=CARTESIAN_POINT ( 'NONE',  ( -5.385316468750001029, -28.88020833299193768, -3.109213912904136734 ) ) ;
#7615=ORIENTED_EDGE ( 'NONE', *, *, #3389, .T. ) ;
#7618=CARTESIAN_POINT ( 'NONE',  ( -3.807688866302469071E-16, -28.67187499965860198, -6.218427825808274356 ) ) ;
#7619=ORIENTED_EDGE ( 'NONE', *, *, #5310, .T. ) ;
#7620=CARTESIAN_POINT ( 'NONE',  ( 5.385316468750001029, -27.72395833299193413, 3.109213912904134958 ) ) ;
#7625=AXIS2_PLACEMENT_3D ( 'NONE', #6420, #8487, #7082 ) ;
#7629=CARTESIAN_POINT ( 'NONE',  ( 2.692658234374998738, -28.91145833299193413, -4.663820869356206877 ) ) ;
#7631=CARTESIAN_POINT ( 'NONE',  ( -6.972266317189433020E-16, -28.49999999931720041, -5.250000000000000000 ) ) ;
#7633=CARTESIAN_POINT ( 'NONE',  ( 2.692658234374998738, -27.19270833299193413, -4.663820869356206877 ) ) ;
#7635=CYLINDRICAL_SURFACE ( 'NONE', #785, 5.250000000000000000 ) ;
#7638=ORIENTED_EDGE ( 'NONE', *, *, #8052, .T. ) ;
#7640=CARTESIAN_POINT ( 'NONE',  ( 5.250000000000000000, -28.37500000000000000, -6.429395695523604153E-16 ) ) ;
#7643=CARTESIAN_POINT ( 'NONE',  ( 1.045839947578414884E-14, -28.06249999999999289, -5.250000000000000000 ) ) ;
#7645=CARTESIAN_POINT ( 'NONE',  ( 0.000000000000000000, -27.00000000000000000, 0.000000000000000000 ) ) ;
#7651=( BOUNDED_CURVE ( )  B_SPLINE_CURVE ( 2, ( #7994, #7204, #829, #6684, #1622, #7389, #8737, #1013, #2981 ),
 .UNSPECIFIED., .F., .F. ) 
 B_SPLINE_CURVE_WITH_KNOTS ( ( 3, 2, 2, 2, 3 ),
 ( 0.6041666666666667407, 0.6111111111111111605, 0.6250000000000000000, 0.6388888888888888395, 0.6458333333333333703 ),
 .UNSPECIFIED. ) 
 CURVE ( )  GEOMETRIC_REPRESENTATION_ITEM ( )  RATIONAL_B_SPLINE_CURVE ( ( 0.9330127018922192983, 0.9330127018922198534, 1.000000000000000000, 0.8660254037844387076, 1.000000000000000000, 0.8660254037844387076, 1.000000000000000000, 0.9330127018922187432, 0.9330127018922192983 ) ) 
 REPRESENTATION_ITEM ( '' )  );
#7652=EDGE_CURVE ( 'NONE', #3243, #2470, #685, .T. ) ;
#7653=FACE_OUTER_BOUND ( 'NONE', #2615, .T. ) ;
#7654=CARTESIAN_POINT ( 'NONE',  ( -5.249999999999999112, -29.41666666598387181, 3.031088913245538308 ) ) ;
#7655=CARTESIAN_POINT ( 'NONE',  ( 5.385316468750001029, -29.75520833299193413, 3.109213912904134958 ) ) ;
#7657=CARTESIAN_POINT ( 'NONE',  ( -3.807688866302469071E-16, -29.17187499965859843, -6.218427825808274356 ) ) ;
#7663=CARTESIAN_POINT ( 'NONE',  ( -3.807688866302469071E-16, -29.17187499965859843, -6.218427825808274356 ) ) ;
#7665=CARTESIAN_POINT ( 'NONE',  ( -5.385316468750000141, -29.82812499965859843, 0.000000000000000000 ) ) ;
#7667=CARTESIAN_POINT ( 'NONE',  ( 0.000000000000000000, -27.00000000000000000, 0.000000000000000000 ) ) ;
#7669=DIRECTION ( 'NONE',  ( 0.000000000000000000, 0.000000000000000000, -1.000000000000000000 ) ) ;
#7670=CYLINDRICAL_SURFACE ( 'NONE', #5788, 5.250000000000000000 ) ;
#7672=FACE_OUTER_BOUND ( 'NONE', #2068, .T. ) ;
#7674=CARTESIAN_POINT ( 'NONE',  ( -2.692658234374996518, -29.78645833299193413, 4.663820869356208654 ) ) ;
#7675=ADVANCED_FACE ( 'NONE', ( #3023 ), #5846, .F. ) ;
#7677=CARTESIAN_POINT ( 'NONE',  ( 5.250000000000000888, -28.58333333265053611, 3.031088913245533423 ) ) ;
#7678=CARTESIAN_POINT ( 'NONE',  ( -5.385316468749998364, -27.33854166632526628, 3.109213912904140287 ) ) ;
#7682=ORIENTED_EDGE ( 'NONE', *, *, #5379, .T. ) ;
#7683=CARTESIAN_POINT ( 'NONE',  ( 1.113604000661152470E-15, -28.68750000000000000, 6.062177826491070398 ) ) ;
#7687=DIRECTION ( 'NONE',  ( 0.000000000000000000, 0.000000000000000000, -1.000000000000000000 ) ) ;
#7693=DIRECTION ( 'NONE',  ( 0.000000000000000000, -1.000000000000000000, 0.000000000000000000 ) ) ;
#7694=CARTESIAN_POINT ( 'NONE',  ( 5.250000000000000000, -29.06249999931720396, -6.429395695523604153E-16 ) ) ;
#7696=CARTESIAN_POINT ( 'NONE',  ( -2.625000000000000444, -27.22916666598386826, -4.546633369868303021 ) ) ;
#7702=( BOUNDED_CURVE ( )  B_SPLINE_CURVE ( 2, ( #7608, #3891, #8810, #1795, #4029, #3194, #3285, #2592, #6665 ),
 .UNSPECIFIED., .F., .F. ) 
 B_SPLINE_CURVE_WITH_KNOTS ( ( 3, 2, 2, 2, 3 ),
 ( 0.2708333333333333703, 0.2777777777777777901, 0.2916666666666666852, 0.3055555555555555802, 0.3125000000000000000 ),
 .UNSPECIFIED. ) 
 CURVE ( )  GEOMETRIC_REPRESENTATION_ITEM ( )  RATIONAL_B_SPLINE_CURVE ( ( 0.9330127018922194093, 0.9330127018922196314, 1.000000000000000000, 0.8660254037844387076, 1.000000000000000000, 0.8660254037844387076, 1.000000000000000000, 0.9330127018922194093, 0.9330127018922194093 ) ) 
 REPRESENTATION_ITEM ( '' )  );
#7703=CARTESIAN_POINT ( 'NONE',  ( 5.385316468750000141, -29.98437499965859843, -6.595110575850215044E-16 ) ) ;
#7704=ADVANCED_FACE ( 'NONE', ( #6127 ), #2696, .F. ) ;
#7706=CARTESIAN_POINT ( 'NONE',  ( 2.692658234374998738, -29.41145833299193413, -4.663820869356206877 ) ) ;
#7711=DIRECTION ( 'NONE',  ( 0.000000000000000000, -1.000000000000000000, 0.000000000000000000 ) ) ;
#7714=AXIS2_PLACEMENT_3D ( 'NONE', #5097, #221, #263 ) ;
#7716=CARTESIAN_POINT ( 'NONE',  ( -5.385316468750000141, -30.10937499965859843, 0.000000000000000000 ) ) ;
#7720=CARTESIAN_POINT ( 'NONE',  ( -3.807688866302469071E-16, -29.14062499965860553, -6.218427825808274356 ) ) ;
#7722=CARTESIAN_POINT ( 'NONE',  ( 5.250000000000000888, -30.08333333265053611, 3.031088913245533423 ) ) ;
#7730=CARTESIAN_POINT ( 'NONE',  ( -3.712013335537174572E-16, -29.56250000000000000, -6.062177826491070398 ) ) ;
#7736=DIRECTION ( 'NONE',  ( 0.000000000000000000, -0.000000000000000000, -1.000000000000000000 ) ) ;
#7739=CARTESIAN_POINT ( 'NONE',  ( 6.429395695523604153E-16, -27.00000000000000000, 5.250000000000000000 ) ) ;
#7743=CARTESIAN_POINT ( 'NONE',  ( 5.250000000000000888, -29.58333333265053611, 3.031088913245532979 ) ) ;
#7747=ORIENTED_EDGE ( 'NONE', *, *, #1863, .F. ) ;
#7749=CARTESIAN_POINT ( 'NONE',  ( -5.249999999999997335, -29.66666666598386826, 3.031088913245538308 ) ) ;
#7753=CARTESIAN_POINT ( 'NONE',  ( -5.385316468749998364, -29.80729166632526628, 3.109213912904140287 ) ) ;
#7762=CARTESIAN_POINT ( 'NONE',  ( -5.250000000000000000, -28.68749999931720396, 0.000000000000000000 ) ) ;
#7766=CARTESIAN_POINT ( 'NONE',  ( -3.807688866302469071E-16, -27.17187499965860198, -6.218427825808274356 ) ) ;
#7772=ORIENTED_EDGE ( 'NONE', *, *, #2843, .T. ) ;
#7775=CARTESIAN_POINT ( 'NONE',  ( -2.625000000000000444, -29.54166666666666785, -4.546633369868303021 ) ) ;
#7782=( BOUNDED_SURFACE ( )  B_SPLINE_SURFACE ( 1, 2, ( 
 ( #5760, #7116, #6604, #2233, #4467, #7957, #233, #6554, #184, #5108, #5812, #5058, #49, #3633, #5904, #8743, #5858, #6455, #7911, #7821, #4376, #3586, #6410, #7208, #5715, #5008, #137, #3678, #6500, #2988, #8650, #4651, #1725, #8146, #1676, #6691, #1020, #3915, #5295, #1072, #3821, #5206, #3870, #6739, #370, #321, #6787, #8835, #7447, #4609, #3173, #7349, #1163, #7397, #5996, #1773, #3129, #5342, #2471, #8048, #4562, #275, #3218, #7494, #413, #6038, #4007, #8791, #1119, #2377, #8875, #6841, #2516, #3261, #3961, #8191, #1820, #6089, #2422, #3310, #8922, #2571, #5389, #8240, #4697, #4520, #5252, #1874, #975, #8097, #7537, #465, #5952, #6141, #6646, #4741, #2093, #3405, #8420, #7720, #2047, #4832, #8970, #3359, #9066, #4232, #7063, #4054, #9110, #2755, #3490, #604, #8332, #6234, #7588, #8282, #1214, #4918, #516, #3448, #6274, #6189, #687, #6933, #9017, #3533, #1348, #2663, #1389, #2706, #2620, #7019, #6889, #4873, #6975, #2799, #5485, #5576, #644, #4186, #5535, #6315, #1917, #5437, #8378 ),
 ( #9151, #1963, #4789, #7766, #7633, #5617, #2007, #8465, #1261, #4100, #561, #7678, #1300, #4142, #2400, #6447, #4274, #5706, #2845, #3154, #5972, #2451, #7107, #8769, #4999, #5277, #778, #4366, #8121, #8074, #39, #5929, #3104, #4319, #5664, #1751, #3625, #300, #253, #998, #5229, #1703, #6492, #7200, #7155, #1430, #8550, #4586, #8814, #4541, #2889, #81, #7373, #2178, #7424, #8510, #8593, #2931, #3578, #1047, #3844, #730, #6357, #5752, #4868, #6669, #6403, #2136, #824, #4958, #7855, #3667, #7813, #1476, #2222, #5048, #7903, #1522, #7515, #347, #491, #1189, #6914, #6117, #8993, #7612, #8308, #4678, #2495, #8946, #538, #6714, #2598, #4078, #4768, #6019, #1144, #3379, #6167, #7657, #3198, #2641, #5415, #8264, #2545, #1895, #7563, #6212, #1236, #9041, #4632, #8856, #442, #4722, #7470, #1099, #3987, #3289, #2683, #1798, #8899, #3895, #6816, #6065, #5317, #4033, #8170, #5513, #394, #8356, #3939, #5462, #6766, #1981, #4812, #3241, #5368, #8217, #1939, #1851, #6867, #3338, #706, #1411, #6334 ) ),
 .UNSPECIFIED., .F., .F., .T. ) 
 B_SPLINE_SURFACE_WITH_KNOTS ( ( 2, 2 ),
 ( 3, 2, 2, 2, 2, 2, 2, 2, 2, 2, 2, 2, 2, 2, 2, 2, 2, 2, 2, 2, 2, 2, 2, 2, 2, 2, 2, 2, 2, 2, 2, 2, 2, 2, 2, 2, 2, 2, 2, 2, 2, 2, 2, 2, 2, 2, 2, 2, 2, 2, 2, 2, 2, 2, 2, 2, 2, 2, 2, 2, 2, 2, 2, 2, 2, 2, 2, 2, 2, 2, 2, 2, 3 ),
 ( 0.000000000000000000, 1.000000000000000000 ),
 ( 0.000000000000000000, 0.01388888888888888812, 0.02777777777777777624, 0.04166666666666666435, 0.05555555555555555247, 0.06944444444444444753, 0.08333333333333332871, 0.09722222222222222376, 0.1111111111111111049, 0.1250000000000000000, 0.1388888888888888951, 0.1527777777777777901, 0.1666666666666666574, 0.1805555555555555525, 0.1944444444444444475, 0.2083333333333333426, 0.2222222222222222099, 0.2361111111111111049, 0.2500000000000000000, 0.2638888888888888951, 0.2777777777777777901, 0.2916666666666666852, 0.3055555555555555802, 0.3194444444444444198, 0.3333333333333333148, 0.3472222222222222099, 0.3611111111111111049, 0.3750000000000000000, 0.3888888888888888951, 0.4027777777777777901, 0.4166666666666666852, 0.4305555555555555802, 0.4444444444444444198, 0.4583333333333333148, 0.4722222222222222099, 0.4861111111111111049, 0.5000000000000000000, 0.5138888888888888395, 0.5277777777777777901, 0.5416666666666666297, 0.5555555555555555802, 0.5694444444444444198, 0.5833333333333333703, 0.5972222222222222099, 0.6111111111111111605, 0.6250000000000000000, 0.6388888888888888395, 0.6527777777777777901, 0.6666666666666666297, 0.6805555555555555802, 0.6944444444444444198, 0.7083333333333333703, 0.7222222222222222099, 0.7361111111111111605, 0.7500000000000000000, 0.7638888888888888395, 0.7777777777777777901, 0.7916666666666666297, 0.8055555555555555802, 0.8194444444444444198, 0.8333333333333333703, 0.8472222222222222099, 0.8611111111111111605, 0.8750000000000000000, 0.8888888888888888395, 0.9027777777777777901, 0.9166666666666666297, 0.9305555555555555802, 0.9444444444444444198, 0.9583333333333333703, 0.9722222222222222099, 0.9861111111111111605, 1.000000000000000000 ),
 .UNSPECIFIED. ) 
 GEOMETRIC_REPRESENTATION_ITEM ( )  RATIONAL_B_SPLINE_SURFACE ( (
 ( 1.000000000000000000, 0.8660254037844387076, 1.000000000000000000, 0.8660254037844387076, 1.000000000000000000, 0.8660254037844387076, 1.000000000000000000, 0.8660254037844387076, 1.000000000000000000, 0.8660254037844387076, 1.000000000000000000, 0.8660254037844387076, 1.000000000000000000, 0.8660254037844387076, 1.000000000000000000, 0.8660254037844387076, 1.000000000000000000, 0.8660254037844387076, 1.000000000000000000, 0.8660254037844387076, 1.000000000000000000, 0.8660254037844387076, 1.000000000000000000, 0.8660254037844387076, 1.000000000000000000, 0.8660254037844387076, 1.000000000000000000, 0.8660254037844387076, 1.000000000000000000, 0.8660254037844387076, 1.000000000000000000, 0.8660254037844387076, 1.000000000000000000, 0.8660254037844387076, 1.000000000000000000, 0.8660254037844387076, 1.000000000000000000, 0.8660254037844387076, 1.000000000000000000, 0.8660254037844387076, 1.000000000000000000, 0.8660254037844387076, 1.000000000000000000, 0.8660254037844387076, 1.000000000000000000, 0.8660254037844387076, 1.000000000000000000, 0.8660254037844387076, 1.000000000000000000, 0.8660254037844387076, 1.000000000000000000, 0.8660254037844387076, 1.000000000000000000, 0.8660254037844387076, 1.000000000000000000, 0.8660254037844387076, 1.000000000000000000, 0.8660254037844387076, 1.000000000000000000, 0.8660254037844387076, 1.000000000000000000, 0.8660254037844387076, 1.000000000000000000, 0.8660254037844387076, 1.000000000000000000, 0.8660254037844387076, 1.000000000000000000, 0.8660254037844387076, 1.000000000000000000, 0.8660254037844387076, 1.000000000000000000, 0.8660254037844387076, 1.000000000000000000, 0.8660254037844387076, 1.000000000000000000, 0.8660254037844387076, 1.000000000000000000, 0.8660254037844387076, 1.000000000000000000, 0.8660254037844387076, 1.000000000000000000, 0.8660254037844387076, 1.000000000000000000, 0.8660254037844387076, 1.000000000000000000, 0.8660254037844387076, 1.000000000000000000, 0.8660254037844387076, 1.000000000000000000, 0.8660254037844387076, 1.000000000000000000, 0.8660254037844387076, 1.000000000000000000, 0.8660254037844387076, 1.000000000000000000, 0.8660254037844387076, 1.000000000000000000, 0.8660254037844387076, 1.000000000000000000, 0.8660254037844387076, 1.000000000000000000, 0.8660254037844387076, 1.000000000000000000, 0.8660254037844387076, 1.000000000000000000, 0.8660254037844387076, 1.000000000000000000, 0.8660254037844387076, 1.000000000000000000, 0.8660254037844387076, 1.000000000000000000, 0.8660254037844387076, 1.000000000000000000, 0.8660254037844387076, 1.000000000000000000, 0.8660254037844387076, 1.000000000000000000, 0.8660254037844387076, 1.000000000000000000, 0.8660254037844387076, 1.000000000000000000, 0.8660254037844387076, 1.000000000000000000, 0.8660254037844387076, 1.000000000000000000, 0.8660254037844387076, 1.000000000000000000, 0.8660254037844387076, 1.000000000000000000, 0.8660254037844387076, 1.000000000000000000, 0.8660254037844387076, 1.000000000000000000, 0.8660254037844387076, 1.000000000000000000, 0.8660254037844387076, 1.000000000000000000, 0.8660254037844387076, 1.000000000000000000, 0.8660254037844387076, 1.000000000000000000, 0.8660254037844387076, 1.000000000000000000, 0.8660254037844387076, 1.000000000000000000),
 ( 1.000000000000000000, 0.8660254037844387076, 1.000000000000000000, 0.8660254037844387076, 1.000000000000000000, 0.8660254037844387076, 1.000000000000000000, 0.8660254037844387076, 1.000000000000000000, 0.8660254037844387076, 1.000000000000000000, 0.8660254037844387076, 1.000000000000000000, 0.8660254037844387076, 1.000000000000000000, 0.8660254037844387076, 1.000000000000000000, 0.8660254037844387076, 1.000000000000000000, 0.8660254037844387076, 1.000000000000000000, 0.8660254037844387076, 1.000000000000000000, 0.8660254037844387076, 1.000000000000000000, 0.8660254037844387076, 1.000000000000000000, 0.8660254037844387076, 1.000000000000000000, 0.8660254037844387076, 1.000000000000000000, 0.8660254037844387076, 1.000000000000000000, 0.8660254037844387076, 1.000000000000000000, 0.8660254037844387076, 1.000000000000000000, 0.8660254037844387076, 1.000000000000000000, 0.8660254037844387076, 1.000000000000000000, 0.8660254037844387076, 1.000000000000000000, 0.8660254037844387076, 1.000000000000000000, 0.8660254037844387076, 1.000000000000000000, 0.8660254037844387076, 1.000000000000000000, 0.8660254037844387076, 1.000000000000000000, 0.8660254037844387076, 1.000000000000000000, 0.8660254037844387076, 1.000000000000000000, 0.8660254037844387076, 1.000000000000000000, 0.8660254037844387076, 1.000000000000000000, 0.8660254037844387076, 1.000000000000000000, 0.8660254037844387076, 1.000000000000000000, 0.8660254037844387076, 1.000000000000000000, 0.8660254037844387076, 1.000000000000000000, 0.8660254037844387076, 1.000000000000000000, 0.8660254037844387076, 1.000000000000000000, 0.8660254037844387076, 1.000000000000000000, 0.8660254037844387076, 1.000000000000000000, 0.8660254037844387076, 1.000000000000000000, 0.8660254037844387076, 1.000000000000000000, 0.8660254037844387076, 1.000000000000000000, 0.8660254037844387076, 1.000000000000000000, 0.8660254037844387076, 1.000000000000000000, 0.8660254037844387076, 1.000000000000000000, 0.8660254037844387076, 1.000000000000000000, 0.8660254037844387076, 1.000000000000000000, 0.8660254037844387076, 1.000000000000000000, 0.8660254037844387076, 1.000000000000000000, 0.8660254037844387076, 1.000000000000000000, 0.8660254037844387076, 1.000000000000000000, 0.8660254037844387076, 1.000000000000000000, 0.8660254037844387076, 1.000000000000000000, 0.8660254037844387076, 1.000000000000000000, 0.8660254037844387076, 1.000000000000000000, 0.8660254037844387076, 1.000000000000000000, 0.8660254037844387076, 1.000000000000000000, 0.8660254037844387076, 1.000000000000000000, 0.8660254037844387076, 1.000000000000000000, 0.8660254037844387076, 1.000000000000000000, 0.8660254037844387076, 1.000000000000000000, 0.8660254037844387076, 1.000000000000000000, 0.8660254037844387076, 1.000000000000000000, 0.8660254037844387076, 1.000000000000000000, 0.8660254037844387076, 1.000000000000000000, 0.8660254037844387076, 1.000000000000000000, 0.8660254037844387076, 1.000000000000000000, 0.8660254037844387076, 1.000000000000000000, 0.8660254037844387076, 1.000000000000000000, 0.8660254037844387076, 1.000000000000000000, 0.8660254037844387076, 1.000000000000000000, 0.8660254037844387076, 1.000000000000000000, 0.8660254037844387076, 1.000000000000000000, 0.8660254037844387076, 1.000000000000000000) ) ) 
 REPRESENTATION_ITEM ( '' )  SURFACE ( )  );
#7788=DIRECTION ( 'NONE',  ( 0.000000000000000000, -1.000000000000000000, 0.000000000000000000 ) ) ;
#7789=EDGE_CURVE ( 'NONE', #2627, #8711, #5378, .T. ) ;
#7790=CARTESIAN_POINT ( 'NONE',  ( 2.625000000000002220, -29.10416666598386826, 4.546633369868302132 ) ) ;
#7791=DIRECTION ( 'NONE',  ( 0.000000000000000000, -1.000000000000000000, 0.000000000000000000 ) ) ;
#7793=CARTESIAN_POINT ( 'NONE',  ( 2.161402558328724325E-14, -28.81250000000000000, -5.250000000000000000 ) ) ;
#7801=CARTESIAN_POINT ( 'NONE',  ( 5.385316468749999252, -29.93229166632526983, -3.109213912904138954 ) ) ;
#7804=ORIENTED_EDGE ( 'NONE', *, *, #8959, .F. ) ;
#7805=CARTESIAN_POINT ( 'NONE',  ( -2.033577675846918216E-14, -29.12499999931720751, 5.250000000000000888 ) ) ;
#7807=CARTESIAN_POINT ( 'NONE',  ( 1.406733260263395735, -27.36383544963256753, 5.250000000000000000 ) ) ;
#7812=CARTESIAN_POINT ( 'NONE',  ( 1.406733260263395735, -28.67633545031537068, 5.250000000000000000 ) ) ;
#7813=CARTESIAN_POINT ( 'NONE',  ( -5.385316468750000141, -28.60937499965860198, 0.000000000000000000 ) ) ;
#7819=CARTESIAN_POINT ( 'NONE',  ( -5.385316468749998364, -27.30729166632526983, 3.109213912904140287 ) ) ;
#7820=VERTEX_POINT ( 'NONE', #3300 ) ;
#7821=CARTESIAN_POINT ( 'NONE',  ( 5.385316468750001029, -27.47395833299193413, 3.109213912904135846 ) ) ;
#7828=CARTESIAN_POINT ( 'NONE',  ( -2.624999999999996891, -29.89583333265053611, 4.546633369868304797 ) ) ;
#7839=ORIENTED_EDGE ( 'NONE', *, *, #7269, .T. ) ;
#7841=ORIENTED_EDGE ( 'NONE', *, *, #8041, .T. ) ;
#7842=CARTESIAN_POINT ( 'NONE',  ( -5.385316468750000141, -29.57812499965859843, 0.000000000000000000 ) ) ;
#7844=CARTESIAN_POINT ( 'NONE',  ( 1.975475456537005874E-15, -28.87499999931720396, 5.249999999999999112 ) ) ;
#7845=ORIENTED_EDGE ( 'NONE', *, *, #6337, .T. ) ;
#7848=DIRECTION ( 'NONE',  ( 0.000000000000000000, -1.000000000000000000, 0.000000000000000000 ) ) ;
#7854=CARTESIAN_POINT ( 'NONE',  ( 5.250000000000000000, -28.62500000000000000, -6.429395695523604153E-16 ) ) ;
#7855=CARTESIAN_POINT ( 'NONE',  ( -2.692658234374996518, -28.56770833299193413, 4.663820869356208654 ) ) ;
#7858=AXIS2_PLACEMENT_3D ( 'NONE', #2022, #7080, #3422 ) ;
#7862=CARTESIAN_POINT ( 'NONE',  ( 2.625000000000002220, -29.91666666666666785, 4.546633369868302132 ) ) ;
#7864=CARTESIAN_POINT ( 'NONE',  ( -1.406733260263391960, -27.19866454968463287, 5.250000000000000000 ) ) ;
#7868=CARTESIAN_POINT ( 'NONE',  ( 5.250000000000000000, -29.37500000000000000, -6.429395695523604153E-16 ) ) ;
#7878=CARTESIAN_POINT ( 'NONE',  ( 1.045839947578414884E-14, -27.81249999999999289, -5.250000000000000000 ) ) ;
#7886=EDGE_CURVE ( 'NONE', #8948, #4503, #6364, .T. ) ;
#7890=CARTESIAN_POINT ( 'NONE',  ( -3.807688866302469071E-16, -27.92187499965860198, -6.218427825808274356 ) ) ;
#7893=VECTOR ( 'NONE', #1336, 1000.000000000000000 ) ;
#7894=ORIENTED_EDGE ( 'NONE', *, *, #2128, .T. ) ;
#7897=CARTESIAN_POINT ( 'NONE',  ( -2.692658234375000514, -27.15104166632526628, -4.663820869356205989 ) ) ;
#7900=CARTESIAN_POINT ( 'NONE',  ( -5.385316468750000141, -27.07812499965860198, 0.000000000000000000 ) ) ;
#7903=CARTESIAN_POINT ( 'NONE',  ( 2.692658234374998738, -28.69270833299193413, -4.663820869356206877 ) ) ;
#7907=CARTESIAN_POINT ( 'NONE',  ( 1.406733260263395735, -29.61383544963256753, 5.250000000000000000 ) ) ;
#7908=ORIENTED_EDGE ( 'NONE', *, *, #9001, .T. ) ;
#7909=CARTESIAN_POINT ( 'NONE',  ( -5.249999999999999112, -29.97916666666666430, 3.031088913245538308 ) ) ;
#7911=CARTESIAN_POINT ( 'NONE',  ( 5.385316468750000141, -27.45312499965860198, -6.595110575850215044E-16 ) ) ;
#7915=CARTESIAN_POINT ( 'NONE',  ( 1.975475456537005874E-15, -29.43750000000000000, 5.250000000000000000 ) ) ;
#7923=CARTESIAN_POINT ( 'NONE',  ( -9.180150650966086169E-15, -28.18749999999999645, 5.250000000000000000 ) ) ;
#7927=ORIENTED_EDGE ( 'NONE', *, *, #4524, .T. ) ;
#7928=CARTESIAN_POINT ( 'NONE',  ( 1.045839947578414884E-14, -27.99999999931720041, -5.250000000000000000 ) ) ;
#7932=AXIS2_PLACEMENT_3D ( 'NONE', #8367, #8497, #6433 ) ;
#7936=CARTESIAN_POINT ( 'NONE',  ( -2.692658234374996518, -27.31770833299193413, 4.663820869356208654 ) ) ;
#7938=CARTESIAN_POINT ( 'NONE',  ( 1.406733260263385521, -29.36383544963257108, 5.250000000000006217 ) ) ;
#7939=ORIENTED_EDGE ( 'NONE', *, *, #8173, .T. ) ;
#7940=CARTESIAN_POINT ( 'NONE',  ( -2.624999999999996891, -27.89583333265053255, 4.546633369868304797 ) ) ;
#7942=CARTESIAN_POINT ( 'NONE',  ( -5.385316468750000141, -28.35937499965860198, 0.000000000000000000 ) ) ;
#7945=CARTESIAN_POINT ( 'NONE',  ( -5.385316468750001029, -27.09895833299193413, -3.109213912904136734 ) ) ;
#7947=CARTESIAN_POINT ( 'NONE',  ( -5.249999999999999112, -29.45833333265053611, -3.031088913245534755 ) ) ;
#7949=CARTESIAN_POINT ( 'NONE',  ( -5.250000000000000000, -28.45833333265053611, -3.031088913245534755 ) ) ;
#7952=ORIENTED_EDGE ( 'NONE', *, *, #4703, .T. ) ;
#7953=CARTESIAN_POINT ( 'NONE',  ( -3.807688866302469071E-16, -27.64062499965859843, -6.218427825808274356 ) ) ;
#7955=CARTESIAN_POINT ( 'NONE',  ( 0.000000000000000000, -27.00000000000000000, -6.250000000000000000 ) ) ;
#7956=ORIENTED_EDGE ( 'NONE', *, *, #4233, .F. ) ;
#7957=CARTESIAN_POINT ( 'NONE',  ( 5.385316468749999252, -27.18229166632526628, -3.109213912904139399 ) ) ;
#7959=ORIENTED_EDGE ( 'NONE', *, *, #4485, .F. ) ;
#7962=CARTESIAN_POINT ( 'NONE',  ( -5.249999999999999112, -27.22916666666666430, 3.031088913245538308 ) ) ;
#7967=CARTESIAN_POINT ( 'NONE',  ( -5.249999999999999112, -27.77083333333333215, -3.031088913245534755 ) ) ;
#7970=EDGE_LOOP ( 'NONE', ( #788, #715, #7772, #6773 ) ) ;
#7971=CARTESIAN_POINT ( 'NONE',  ( 0.000000000000000000, -27.00000000000000000, -5.250000000000000000 ) ) ;
#7974=CARTESIAN_POINT ( 'NONE',  ( 2.625000000000002220, -29.66666666666666785, 4.546633369868302132 ) ) ;
#7975=CARTESIAN_POINT ( 'NONE',  ( 2.625000000000002220, -28.16666666666666785, 4.546633369868302132 ) ) ;
#7980=LINE ( 'NONE', #255, #1786 ) ;
#7981=CARTESIAN_POINT ( 'NONE',  ( -5.385316468749998364, -28.58854166632526983, 3.109213912904140287 ) ) ;
#7984=CARTESIAN_POINT ( 'NONE',  ( 5.385316468749999252, -27.43229166632526628, -3.109213912904138954 ) ) ;
#7986=CARTESIAN_POINT ( 'NONE',  ( -5.250000000000000000, -29.43749999931720041, 0.000000000000000000 ) ) ;
#7989=CARTESIAN_POINT ( 'NONE',  ( -5.250000000000000000, -27.95833333265052900, -3.031088913245534755 ) ) ;
#7994=CARTESIAN_POINT ( 'NONE',  ( 2.161402558328724325E-14, -28.99999999931720751, -5.250000000000000000 ) ) ;
#7997=CARTESIAN_POINT ( 'NONE',  ( -3.807688866302469071E-16, -28.64062499965860198, -6.218427825808274356 ) ) ;
#8005=APPLICATION_CONTEXT ( 'automotive_design' ) ;
#8008=CARTESIAN_POINT ( 'NONE',  ( -5.385316468750000141, -27.07812499965860198, 0.000000000000000000 ) ) ;
#8014=VERTEX_POINT ( 'NONE', #7144 ) ;
#8023=DIRECTION ( 'NONE',  ( 0.000000000000000000, 0.000000000000000000, -1.000000000000000000 ) ) ;
#8029=CARTESIAN_POINT ( 'NONE',  ( 5.385316468750001029, -27.50520833299193768, 3.109213912904135846 ) ) ;
#8031=ORIENTED_EDGE ( 'NONE', *, *, #2513, .T. ) ;
#8032=CARTESIAN_POINT ( 'NONE',  ( -5.385316468750001029, -27.34895833299193413, -3.109213912904136734 ) ) ;
#8038=CARTESIAN_POINT ( 'NONE',  ( 2.624999999999998668, -27.77083333265053255, -4.546633369868303021 ) ) ;
#8041=EDGE_CURVE ( 'NONE', #2470, #6852, #4860, .T. ) ;
#8044=CARTESIAN_POINT ( 'NONE',  ( 2.692658234374998738, -28.16145833299193413, -4.663820869356206877 ) ) ;
#8048=CARTESIAN_POINT ( 'NONE',  ( -5.385316468749998364, -28.30729166632526628, 3.109213912904140287 ) ) ;
#8050=VERTEX_POINT ( 'NONE', #2037 ) ;
#8052=EDGE_CURVE ( 'NONE', #105, #4617, #2078, .T. ) ;
#8056=CARTESIAN_POINT ( 'NONE',  ( 2.625000000000002220, -27.41666666666666430, 4.546633369868302132 ) ) ;
#8060=CARTESIAN_POINT ( 'NONE',  ( -1.406733260263397289, -28.19866454968463287, 5.249999999999997335 ) ) ;
#8063=CONICAL_SURFACE ( 'NONE', #3025, 5.257453848358681014, 0.1221730476396033355 ) ;
#8070=CARTESIAN_POINT ( 'NONE',  ( 1.142306659890740623E-15, -27.29687499965859843, 6.218427825808274356 ) ) ;
#8074=CARTESIAN_POINT ( 'NONE',  ( 5.385316468749999252, -27.71354166632526272, -3.109213912904139399 ) ) ;
#8078=( BOUNDED_CURVE ( )  B_SPLINE_CURVE ( 2, ( #7518, #4039, #7567, #2601, #1147, #3990, #5559, #759, #4168 ),
 .UNSPECIFIED., .F., .T. ) 
 B_SPLINE_CURVE_WITH_KNOTS ( ( 3, 2, 2, 2, 3 ),
 ( 0.1458333333333333426, 0.1527777777777777901, 0.1666666666666666574, 0.1805555555555555525, 0.1875000000000000000 ),
 .UNSPECIFIED. ) 
 CURVE ( )  GEOMETRIC_REPRESENTATION_ITEM ( )  RATIONAL_B_SPLINE_CURVE ( ( 0.9330127018922194093, 0.9330127018922194093, 1.000000000000000000, 0.8660254037844387076, 1.000000000000000000, 0.8660254037844387076, 1.000000000000000000, 0.9330127018922194093, 0.9330127018922194093 ) ) 
 REPRESENTATION_ITEM ( '' )  );
#8079=CARTESIAN_POINT ( 'NONE',  ( 2.692658234375002735, -28.27604166632526628, 4.663820869356205101 ) ) ;
#8086=CARTESIAN_POINT ( 'NONE',  ( -2.624999999999996891, -27.39583333265053611, 4.546633369868304797 ) ) ;
#8087=CARTESIAN_POINT ( 'NONE',  ( 5.249999999999999112, -27.60416666666666430, -3.031088913245536975 ) ) ;
#8089=DIRECTION ( 'NONE',  ( 0.000000000000000000, -1.000000000000000000, 0.000000000000000000 ) ) ;
#8092=CARTESIAN_POINT ( 'NONE',  ( -2.692658234375000514, -27.61979166632526628, -4.663820869356205989 ) ) ;
#8095=CARTESIAN_POINT ( 'NONE',  ( -5.249999999999999112, -28.52083333333333215, -3.031088913245534755 ) ) ;
#8097=CARTESIAN_POINT ( 'NONE',  ( 5.385316468749999252, -28.93229166632526628, -3.109213912904139399 ) ) ;
#8099=VERTEX_POINT ( 'NONE', #7844 ) ;
#8113=EDGE_CURVE ( 'NONE', #3780, #2524, #4260, .T. ) ;
#8117=CARTESIAN_POINT ( 'NONE',  ( 7.654042494670957606E-16, -27.00000000000000000, 6.250000000000000000 ) ) ;
#8118=CARTESIAN_POINT ( 'NONE',  ( -2.692658234374996518, -28.31770833299193413, 4.663820869356208654 ) ) ;
#8121=CARTESIAN_POINT ( 'NONE',  ( 2.692658234374998738, -27.69270833299193768, -4.663820869356206877 ) ) ;
#8124=CARTESIAN_POINT ( 'NONE',  ( -1.406733260263391960, -27.88616454900183328, 5.250000000000000000 ) ) ;
#8126=CARTESIAN_POINT ( 'NONE',  ( 2.692658234374998738, -27.44270833299193413, -4.663820869356206877 ) ) ;
#8128=VERTEX_POINT ( 'NONE', #8583 ) ;
#8130=CARTESIAN_POINT ( 'NONE',  ( 5.385316468750001029, -28.72395833299193413, 3.109213912904134958 ) ) ;
#8135=CARTESIAN_POINT ( 'NONE',  ( 5.250000000000000888, -27.33333333265053611, 3.031088913245532979 ) ) ;
#8141=CARTESIAN_POINT ( 'NONE',  ( -5.385316468749998364, -28.80729166632526983, 3.109213912904140287 ) ) ;
#8146=CARTESIAN_POINT ( 'NONE',  ( 1.142306659890740623E-15, -27.76562499965860198, 6.218427825808274356 ) ) ;
#8151=ORIENTED_EDGE ( 'NONE', *, *, #6449, .F. ) ;
#8155=VECTOR ( 'NONE', #7788, 1000.000000000000000 ) ;
#8159=CARTESIAN_POINT ( 'NONE',  ( 0.000000000000000000, -50.00000000000000000, -3.794308781941904574 ) ) ;
#8168=CARTESIAN_POINT ( 'NONE',  ( 5.385316468750001029, -28.25520833299193413, 3.109213912904134958 ) ) ;
#8170=CARTESIAN_POINT ( 'NONE',  ( 5.385316468750000141, -29.73437499965859843, -6.595110575850215044E-16 ) ) ;
#8172=ORIENTED_EDGE ( 'NONE', *, *, #6696, .F. ) ;
#8173=EDGE_CURVE ( 'NONE', #2212, #3243, #2291, .T. ) ;
#8177=CARTESIAN_POINT ( 'NONE',  ( -5.385316468749998364, -29.58854166632527694, 3.109213912904140287 ) ) ;
#8179=CARTESIAN_POINT ( 'NONE',  ( 5.385316468750000141, -27.70312499965860198, -6.595110575850215044E-16 ) ) ;
#8183=CARTESIAN_POINT ( 'NONE',  ( -9.180150650966086169E-15, -28.37499999931720041, 5.250000000000000000 ) ) ;
#8184=CARTESIAN_POINT ( 'NONE',  ( 0.000000000000000000, -27.00000000000000000, 0.000000000000000000 ) ) ;
#8188=CARTESIAN_POINT ( 'NONE',  ( 5.385316468749999252, -29.68229166632526983, -3.109213912904139399 ) ) ;
#8190=CARTESIAN_POINT ( 'NONE',  ( -6.972266317189433020E-16, -29.06249999999999645, -5.249999999999999112 ) ) ;
#8191=CARTESIAN_POINT ( 'NONE',  ( -3.807688866302469071E-16, -28.64062499965860198, -6.218427825808274356 ) ) ;
#8194=ORIENTED_EDGE ( 'NONE', *, *, #2445, .F. ) ;
#8196=FACE_OUTER_BOUND ( 'NONE', #4424, .T. ) ;
#8199=CARTESIAN_POINT ( 'NONE',  ( 2.624999999999998668, -28.58333333333333215, -4.546633369868303021 ) ) ;
#8210=ORIENTED_EDGE ( 'NONE', *, *, #8113, .F. ) ;
#8212=ADVANCED_FACE ( 'NONE', ( #5786 ), #4593, .F. ) ;
#8213=CARTESIAN_POINT ( 'NONE',  ( 1.142306659890740623E-15, -28.54687499965860198, 6.218427825808274356 ) ) ;
#8215=CARTESIAN_POINT ( 'NONE',  ( 2.692658234375002735, -29.77604166632526983, 4.663820869356205101 ) ) ;
#8217=CARTESIAN_POINT ( 'NONE',  ( 5.385316468749999252, -29.96354166632526628, -3.109213912904139399 ) ) ;
#8219=CIRCLE ( 'NONE', #3469, 5.250000000000000000 ) ;
#8221=CARTESIAN_POINT ( 'NONE',  ( 7.654042494670957606E-16, -30.00000000000000000, 6.250000000000000000 ) ) ;
#8223=CARTESIAN_POINT ( 'NONE',  ( -5.385316468750001029, -29.13020833299193058, -3.109213912904136734 ) ) ;
#8227=CARTESIAN_POINT ( 'NONE',  ( 5.385316468750000141, -28.70312499965860198, -6.595110575850215044E-16 ) ) ;
#8230=AXIS2_PLACEMENT_3D ( 'NONE', #3253, #5527, #7669 ) ;
#8233=CARTESIAN_POINT ( 'NONE',  ( 2.625000000000002220, -27.41666666666666430, 4.546633369868302132 ) ) ;
#8240=CARTESIAN_POINT ( 'NONE',  ( -5.385316468749998364, -28.80729166632526983, 3.109213912904140287 ) ) ;
#8248=( NAMED_UNIT ( * ) PLANE_ANGLE_UNIT ( ) SI_UNIT ( $, .RADIAN. ) );
#8249=CARTESIAN_POINT ( 'NONE',  ( -2.625000000000000444, -29.04166666666666785, -4.546633369868303021 ) ) ;
#8250=ORIENTED_EDGE ( 'NONE', *, *, #5006, .F. ) ;
#8261=CARTESIAN_POINT ( 'NONE',  ( -5.385316468750001029, -29.38020833299193413, -3.109213912904136734 ) ) ;
#8262=CARTESIAN_POINT ( 'NONE',  ( 5.385316468749999252, -29.96354166632527338, -3.109213912904138954 ) ) ;
#8264=CARTESIAN_POINT ( 'NONE',  ( 5.385316468750001029, -29.25520833299193058, 3.109213912904135846 ) ) ;
#8269=CARTESIAN_POINT ( 'NONE',  ( -5.385316468750001029, -28.63020833299193413, -3.109213912904136734 ) ) ;
#8270=ORIENTED_EDGE ( 'NONE', *, *, #6799, .T. ) ;
#8271=CARTESIAN_POINT ( 'NONE',  ( 5.385316468750001029, -27.97395833299193413, 3.109213912904134958 ) ) ;
#8275=CARTESIAN_POINT ( 'NONE',  ( -1.406733260263394625, -28.48883544963257464, -5.250000000000000000 ) ) ;
#8280=CARTESIAN_POINT ( 'NONE',  ( -5.385316468749998364, -29.80729166632526628, 3.109213912904140287 ) ) ;
#8282=CARTESIAN_POINT ( 'NONE',  ( 5.385316468750001029, -29.47395833299193413, 3.109213912904135846 ) ) ;
#8285=ORIENTED_EDGE ( 'NONE', *, *, #4485, .T. ) ;
#8287=DIRECTION ( 'NONE',  ( 0.000000000000000000, -1.000000000000000000, 0.000000000000000000 ) ) ;
#8292=CARTESIAN_POINT ( 'NONE',  ( -5.249999999999999112, -28.97916666666666430, 3.031088913245538308 ) ) ;
#8293=ORIENTED_EDGE ( 'NONE', *, *, #6301, .T. ) ;
#8299=CARTESIAN_POINT ( 'NONE',  ( -6.972266317189433020E-16, -29.24999999931720396, -5.250000000000000000 ) ) ;
#8305=CARTESIAN_POINT ( 'NONE',  ( -2.692658234375000514, -29.15104166632526983, -4.663820869356205989 ) ) ;
#8307=CARTESIAN_POINT ( 'NONE',  ( 0.000000000000000000, -27.00000000000000000, 0.000000000000000000 ) ) ;
#8308=CARTESIAN_POINT ( 'NONE',  ( -2.692658234375000514, -28.90104166632526983, -4.663820869356205989 ) ) ;
#8315=CARTESIAN_POINT ( 'NONE',  ( -3.807688866302469071E-16, -29.92187499965859843, -6.218427825808274356 ) ) ;
#8318=CARTESIAN_POINT ( 'NONE',  ( 2.692658234374998738, -28.41145833299193413, -4.663820869356206877 ) ) ;
#8322=FACE_OUTER_BOUND ( 'NONE', #7970, .T. ) ;
#8329=CARTESIAN_POINT ( 'NONE',  ( 5.385316468749999252, -28.93229166632526628, -3.109213912904139399 ) ) ;
#8331=CARTESIAN_POINT ( 'NONE',  ( -1.406733260263384411, -29.55133545031537423, -5.250000000000006217 ) ) ;
#8332=CARTESIAN_POINT ( 'NONE',  ( 2.692658234374998738, -29.41145833299193413, -4.663820869356206877 ) ) ;
#8340=SHAPE_REPRESENTATION_RELATIONSHIP ( 'NONE' , 'NONE' ,  #6994, #3635 ) ;
#8341=CARTESIAN_POINT ( 'NONE',  ( -5.250000000000000000, -28.50000000000000000, 0.000000000000000000 ) ) ;
#8346=CARTESIAN_POINT ( 'NONE',  ( 5.249999999999999112, -28.10416666666666785, -3.031088913245536975 ) ) ;
#8348=DIRECTION ( 'NONE',  ( 0.000000000000000000, 0.000000000000000000, -1.000000000000000000 ) ) ;
#8352=CARTESIAN_POINT ( 'NONE',  ( -5.249999999999999112, -28.77083333333333215, -3.031088913245534755 ) ) ;
#8353=CARTESIAN_POINT ( 'NONE',  ( 2.624999999999998668, -28.77083333265053611, -4.546633369868303021 ) ) ;
#8354=CARTESIAN_POINT ( 'NONE',  ( 2.692658234375002735, -30.02604166632526983, 4.663820869356205101 ) ) ;
#8356=CARTESIAN_POINT ( 'NONE',  ( 1.142306659890740623E-15, -29.79687499965859843, 6.218427825808274356 ) ) ;
#8359=ORIENTED_EDGE ( 'NONE', *, *, #8959, .T. ) ;
#8362=ADVANCED_FACE ( 'NONE', ( #6166 ), #2682, .T. ) ;
#8364=CARTESIAN_POINT ( 'NONE',  ( 2.692658234375002735, -29.52604166632526983, 4.663820869356205101 ) ) ;
#8367=CARTESIAN_POINT ( 'NONE',  ( 0.000000000000000000, -27.00000000000000000, 0.000000000000000000 ) ) ;
#8370=CARTESIAN_POINT ( 'NONE',  ( -1.406733260263397289, -28.38616454900183328, 5.249999999999997335 ) ) ;
#8373=VECTOR ( 'NONE', #4711, 1000.000000000000000 ) ;
#8375=CARTESIAN_POINT ( 'NONE',  ( -5.249999999999997335, -28.16666666598386826, 3.031088913245538308 ) ) ;
#8376=CARTESIAN_POINT ( 'NONE',  ( 1.142306659890740623E-15, -29.76562499965859843, 6.218427825808274356 ) ) ;
#8378=CARTESIAN_POINT ( 'NONE',  ( -5.385316468750000141, -30.07812499965859843, 0.000000000000000000 ) ) ;
#8383=( BOUNDED_CURVE ( )  B_SPLINE_CURVE ( 2, ( #8689, #2978, #3719, #8087, #3074, #869, #2320, #8641, #8827 ),
 .UNSPECIFIED., .F., .F. ) 
 B_SPLINE_CURVE_WITH_KNOTS ( ( 3, 2, 2, 2, 3 ),
 ( 0.1875000000000000000, 0.1944444444444444475, 0.2083333333333333426, 0.2222222222222222099, 0.2291666666666666574 ),
 .UNSPECIFIED. ) 
 CURVE ( )  GEOMETRIC_REPRESENTATION_ITEM ( )  RATIONAL_B_SPLINE_CURVE ( ( 0.9330127018922194093, 0.9330127018922194093, 1.000000000000000000, 0.8660254037844387076, 1.000000000000000000, 0.8660254037844387076, 1.000000000000000000, 0.9330127018922194093, 0.9330127018922194093 ) ) 
 REPRESENTATION_ITEM ( '' )  );
#8385=VERTEX_POINT ( 'NONE', #1850 ) ;
#8386=CARTESIAN_POINT ( 'NONE',  ( -5.250000000000000000, -28.02083333333333215, -3.031088913245534755 ) ) ;
#8390=CARTESIAN_POINT ( 'NONE',  ( -1.406733260263402174, -29.94866454968462577, 5.249999999999995559 ) ) ;
#8396=CARTESIAN_POINT ( 'NONE',  ( -1.406733260263402174, -29.19866454968462577, 5.249999999999995559 ) ) ;
#8397=CARTESIAN_POINT ( 'NONE',  ( 5.250000000000000000, -29.29166666598386826, -3.031088913245536531 ) ) ;
#8398=CARTESIAN_POINT ( 'NONE',  ( -5.385316468749998364, -30.08854166632526983, 3.109213912904140287 ) ) ;
#8403=ORIENTED_EDGE ( 'NONE', *, *, #2854, .F. ) ;
#8406=CARTESIAN_POINT ( 'NONE',  ( 2.692658234375002735, -30.02604166632526983, 4.663820869356205101 ) ) ;
#8408=CARTESIAN_POINT ( 'NONE',  ( 2.692658234374998738, -29.16145833299193413, -4.663820869356206877 ) ) ;
#8412=CARTESIAN_POINT ( 'NONE',  ( -5.385316468750000141, -30.07812499965859843, 0.000000000000000000 ) ) ;
#8416=CYLINDRICAL_SURFACE ( 'NONE', #1839, 5.250000000000000000 ) ;
#8417=DIRECTION ( 'NONE',  ( 0.000000000000000000, 0.000000000000000000, -1.000000000000000000 ) ) ;
#8420=CARTESIAN_POINT ( 'NONE',  ( -2.692658234375000514, -29.11979166632526983, -4.663820869356205989 ) ) ;
#8427=CARTESIAN_POINT ( 'NONE',  ( -2.624999999999996891, -29.95833333333333215, 4.546633369868304797 ) ) ;
#8431=CARTESIAN_POINT ( 'NONE',  ( 0.000000000000000000, -30.00000000000000000, 0.000000000000000000 ) ) ;
#8437=CARTESIAN_POINT ( 'NONE',  ( -5.250000000000000000, -29.70833333265053611, -3.031088913245534755 ) ) ;
#8448=ORIENTED_EDGE ( 'NONE', *, *, #5988, .T. ) ;
#8449=CARTESIAN_POINT ( 'NONE',  ( -2.692658234375000514, -29.36979166632526983, -4.663820869356205989 ) ) ;
#8452=DIRECTION ( 'NONE',  ( 0.000000000000000000, -1.000000000000000000, 0.000000000000000000 ) ) ;
#8453=AXIS2_PLACEMENT_3D ( 'NONE', #4141, #1162, #1819 ) ;
#8455=VERTEX_POINT ( 'NONE', #7793 ) ;
#8459=AXIS2_PLACEMENT_3D ( 'NONE', #7667, #7574, #2651 ) ;
#8465=CARTESIAN_POINT ( 'NONE',  ( 5.385316468750001029, -27.25520833299193413, 3.109213912904135846 ) ) ;
#8467=VECTOR ( 'NONE', #5725, 1000.000000000000000 ) ;
#8475=CARTESIAN_POINT ( 'NONE',  ( -3.807688866302469071E-16, -27.14062499965860198, -6.218427825808274356 ) ) ;
#8486=CARTESIAN_POINT ( 'NONE',  ( 5.250000000000000000, -29.56249999931720041, -6.429395695523604153E-16 ) ) ;
#8487=DIRECTION ( 'NONE',  ( 0.000000000000000000, -1.000000000000000000, 0.000000000000000000 ) ) ;
#8493=VECTOR ( 'NONE', #6267, 1000.000000000000000 ) ;
#8497=DIRECTION ( 'NONE',  ( 0.000000000000000000, -1.000000000000000000, 0.000000000000000000 ) ) ;
#8499=DIRECTION ( 'NONE',  ( 0.000000000000000000, -1.000000000000000000, 0.000000000000000000 ) ) ;
#8504=CARTESIAN_POINT ( 'NONE',  ( 0.000000000000000000, -30.00000000000000000, 0.000000000000000000 ) ) ;
#8507=CARTESIAN_POINT ( 'NONE',  ( -5.249999999999997335, -28.66666666598387181, 3.031088913245538308 ) ) ;
#8509=FACE_OUTER_BOUND ( 'NONE', #3651, .T. ) ;
#8510=CARTESIAN_POINT ( 'NONE',  ( 5.385316468750001029, -28.25520833299193413, 3.109213912904135846 ) ) ;
#8515=ORIENTED_EDGE ( 'NONE', *, *, #6771, .T. ) ;
#8518=CARTESIAN_POINT ( 'NONE',  ( 2.625000000000002220, -29.41666666666666785, 4.546633369868302132 ) ) ;
#8522=CARTESIAN_POINT ( 'NONE',  ( 5.250000000000000888, -29.39583333333332860, 3.031088913245533423 ) ) ;
#8526=CARTESIAN_POINT ( 'NONE',  ( -2.625000000000000444, -29.22916666598386826, -4.546633369868303021 ) ) ;
#8533=CARTESIAN_POINT ( 'NONE',  ( -5.249999999999999112, -28.95833333265053611, -3.031088913245534755 ) ) ;
#8538=CARTESIAN_POINT ( 'NONE',  ( -2.692658234375000514, -29.61979166632526983, -4.663820869356205989 ) ) ;
#8541=ORIENTED_EDGE ( 'NONE', *, *, #7167, .T. ) ;
#8542=LINE ( 'NONE', #595, #1492 ) ;
#8550=CARTESIAN_POINT ( 'NONE',  ( -2.692658234374996518, -28.06770833299193413, 4.663820869356208654 ) ) ;
#8556=CARTESIAN_POINT ( 'NONE',  ( -2.625000000000000444, -29.79166666666666785, -4.546633369868303021 ) ) ;
#8557=EDGE_LOOP ( 'NONE', ( #9024, #4444, #7841, #7598 ) ) ;
#8558=FACE_OUTER_BOUND ( 'NONE', #4522, .T. ) ;
#8560=ORIENTED_EDGE ( 'NONE', *, *, #2475, .F. ) ;
#8570=DIRECTION ( 'NONE',  ( 0.8660254037844402619, 0.4999999999999970579, -0.000000000000000000 ) ) ;
#8583=CARTESIAN_POINT ( 'NONE',  ( -6.972266317189433020E-16, -27.74999999931720041, -5.249999999999999112 ) ) ;
#8584=VERTEX_POINT ( 'NONE', #196 ) ;
#8588=CARTESIAN_POINT ( 'NONE',  ( 0.000000000000000000, -30.00000000000000000, -6.250000000000000000 ) ) ;
#8589=AXIS2_PLACEMENT_3D ( 'NONE', #4114, #7693, #4160 ) ;
#8591=( BOUNDED_CURVE ( )  B_SPLINE_CURVE ( 2, ( #660, #6368, #2858, #5719, #7868, #8522, #2150, #7212, #7915 ),
 .UNSPECIFIED., .F., .F. ) 
 B_SPLINE_CURVE_WITH_KNOTS ( ( 3, 2, 2, 2, 3 ),
 ( 0.7708333333333333703, 0.7777777777777777901, 0.7916666666666666297, 0.8055555555555555802, 0.8125000000000000000 ),
 .UNSPECIFIED. ) 
 CURVE ( )  GEOMETRIC_REPRESENTATION_ITEM ( )  RATIONAL_B_SPLINE_CURVE ( ( 0.9330127018922192983, 0.9330127018922198534, 1.000000000000000000, 0.8660254037844387076, 1.000000000000000000, 0.8660254037844387076, 1.000000000000000000, 0.9330127018922194093, 0.9330127018922194093 ) ) 
 REPRESENTATION_ITEM ( '' )  );
#8592=CARTESIAN_POINT ( 'NONE',  ( 5.249999999999999112, -28.60416666666666430, -3.031088913245536975 ) ) ;
#8593=CARTESIAN_POINT ( 'NONE',  ( 2.692658234375002735, -28.27604166632526628, 4.663820869356205101 ) ) ;
#8599=CARTESIAN_POINT ( 'NONE',  ( 1.113604000661152470E-15, -29.18750000000000000, 6.062177826491070398 ) ) ;
#8601=ORIENTED_EDGE ( 'NONE', *, *, #6379, .T. ) ;
#8604=ORIENTED_EDGE ( 'NONE', *, *, #5430, .T. ) ;
#8614=CARTESIAN_POINT ( 'NONE',  ( -1.406733260263402174, -29.88616454900183328, 5.249999999999995559 ) ) ;
#8623=EDGE_LOOP ( 'NONE', ( #1992, #3568, #2867, #5780 ) ) ;
#8624=EDGE_LOOP ( 'NONE', ( #2742, #7615, #2098, #1128 ) ) ;
#8625=CARTESIAN_POINT ( 'NONE',  ( -6.972266317189433020E-16, -29.81250000000000000, -5.250000000000000000 ) ) ;
#8626=CARTESIAN_POINT ( 'NONE',  ( 2.692658234375002735, -27.77604166632526628, 4.663820869356205101 ) ) ;
#8640=CARTESIAN_POINT ( 'NONE',  ( 1.113604000661152470E-15, -28.37499999931720396, 6.062177826491070398 ) ) ;
#8641=CARTESIAN_POINT ( 'NONE',  ( 1.406733260263395735, -27.67633545031536713, 5.250000000000000000 ) ) ;
#8644=CARTESIAN_POINT ( 'NONE',  ( 5.250000000000000000, -29.81249999931720041, -6.429395695523604153E-16 ) ) ;
#8647=CARTESIAN_POINT ( 'NONE',  ( -2.692658234374996518, -28.78645833299193413, 4.663820869356208654 ) ) ;
#8648=CARTESIAN_POINT ( 'NONE',  ( -5.250000000000000000, -28.75000000000000000, 0.000000000000000000 ) ) ;
#8650=CARTESIAN_POINT ( 'NONE',  ( 5.385316468750000141, -27.70312499965860198, -6.595110575850215044E-16 ) ) ;
#8656=VECTOR ( 'NONE', #2238, 1000.000000000000000 ) ;
#8661=EDGE_CURVE ( 'NONE', #3780, #5282, #6683, .T. ) ;
#8662=CARTESIAN_POINT ( 'NONE',  ( -5.250000000000000000, -29.93749999931720041, 0.000000000000000000 ) ) ;
#8667=CARTESIAN_POINT ( 'NONE',  ( 1.975475456537005874E-15, -27.18750000000000000, 5.250000000000000000 ) ) ;
#8670=AXIS2_PLACEMENT_3D ( 'NONE', #2751, #3530, #8417 ) ;
#8671=ORIENTED_EDGE ( 'NONE', *, *, #4211, .T. ) ;
#8672=CARTESIAN_POINT ( 'NONE',  ( 1.406733260263403507, -29.57366454968462932, -5.249999999999994671 ) ) ;
#8673=EDGE_CURVE ( 'NONE', #3243, #7319, #841, .T. ) ;
#8674=CARTESIAN_POINT ( 'NONE',  ( 2.692658234374998738, -27.19270833299193413, -4.663820869356206877 ) ) ;
#8676=ORIENTED_EDGE ( 'NONE', *, *, #1659, .T. ) ;
#8677=ADVANCED_FACE ( 'NONE', ( #8756, #5069 ), #2293, .T. ) ;
#8680=CARTESIAN_POINT ( 'NONE',  ( 1.142306659890740623E-15, -28.29687499965860553, 6.218427825808274356 ) ) ;
#8683=CARTESIAN_POINT ( 'NONE',  ( 1.975475456537005874E-15, -28.87499999931720396, 5.250000000000000000 ) ) ;
#8686=CARTESIAN_POINT ( 'NONE',  ( -5.249999999999997335, -27.41666666598387181, 3.031088913245538308 ) ) ;
#8688=CARTESIAN_POINT ( 'NONE',  ( -2.625000000000000444, -27.97916666598386826, -4.546633369868303021 ) ) ;
#8689=CARTESIAN_POINT ( 'NONE',  ( -6.972266317189433020E-16, -27.56249999999999645, -5.250000000000000000 ) ) ;
#8691=CARTESIAN_POINT ( 'NONE',  ( 2.624999999999998668, -29.52083333265053611, -4.546633369868303021 ) ) ;
#8694=CARTESIAN_POINT ( 'NONE',  ( -5.385316468750001029, -28.09895833299193413, -3.109213912904136734 ) ) ;
#8696=CYLINDRICAL_SURFACE ( 'NONE', #4438, 5.250000000000000000 ) ;
#8705=CARTESIAN_POINT ( 'NONE',  ( -2.033577675846918216E-14, -28.93750000000000000, 5.250000000000000888 ) ) ;
#8708=CARTESIAN_POINT ( 'NONE',  ( -5.249999999999999112, -28.27083333333332860, -3.031088913245534755 ) ) ;
#8710=CARTESIAN_POINT ( 'NONE',  ( 0.000000000000000000, -27.00000000000000000, 0.000000000000000000 ) ) ;
#8711=VERTEX_POINT ( 'NONE', #3091 ) ;
#8715=ORIENTED_EDGE ( 'NONE', *, *, #4351, .F. ) ;
#8716=CARTESIAN_POINT ( 'NONE',  ( -5.249999999999999112, -29.77083333333332860, -3.031088913245534755 ) ) ;
#8717=CARTESIAN_POINT ( 'NONE',  ( -2.692658234374996518, -28.06770833299193413, 4.663820869356208654 ) ) ;
#8725=CARTESIAN_POINT ( 'NONE',  ( 1.142306659890740623E-15, -27.79687499965860198, 6.218427825808274356 ) ) ;
#8727=DIRECTION ( 'NONE',  ( 0.000000000000000000, -1.000000000000000000, 0.000000000000000000 ) ) ;
#8728=CARTESIAN_POINT ( 'NONE',  ( 1.406733260263395735, -28.86383544963257464, 5.250000000000000000 ) ) ;
#8734=CARTESIAN_POINT ( 'NONE',  ( 5.250000000000000000, -28.29166666598387181, -3.031088913245536531 ) ) ;
#8735=CARTESIAN_POINT ( 'NONE',  ( -6.972266317189433020E-16, -27.74999999931720041, -5.250000000000000000 ) ) ;
#8737=CARTESIAN_POINT ( 'NONE',  ( 2.625000000000002220, -29.10416666598386826, 4.546633369868302132 ) ) ;
#8739=CARTESIAN_POINT ( 'NONE',  ( 1.142306659890740623E-15, -28.76562499965860553, 6.218427825808274356 ) ) ;
#8743=CARTESIAN_POINT ( 'NONE',  ( -3.807688866302469071E-16, -27.39062499965860198, -6.218427825808274356 ) ) ;
#8745=VERTEX_POINT ( 'NONE', #1546 ) ;
#8753=CARTESIAN_POINT ( 'NONE',  ( -5.250000000000000000, -27.52083333333333570, -3.031088913245534755 ) ) ;
#8756=FACE_BOUND ( 'NONE', #3798, .T. ) ;
#8757=CARTESIAN_POINT ( 'NONE',  ( -5.249999999999997335, -27.72916666666666430, 3.031088913245538308 ) ) ;
#8762=CARTESIAN_POINT ( 'NONE',  ( -6.972266317189433020E-16, -27.06250000000000000, -5.249999999999999112 ) ) ;
#8766=CARTESIAN_POINT ( 'NONE',  ( -5.385316468750000141, -27.10937499965860198, 0.000000000000000000 ) ) ;
#8768=CARTESIAN_POINT ( 'NONE',  ( 2.624999999999998668, -29.27083333265053611, -4.546633369868303021 ) ) ;
#8769=CARTESIAN_POINT ( 'NONE',  ( -5.385316468749998364, -27.58854166632526983, 3.109213912904140287 ) ) ;
#8772=CARTESIAN_POINT ( 'NONE',  ( 1.406733260263393293, -29.82366454968462932, -5.250000000000000000 ) ) ;
#8774=CARTESIAN_POINT ( 'NONE',  ( -5.385316468750000141, -27.60937499965860198, 0.000000000000000000 ) ) ;
#8776=ORIENTED_EDGE ( 'NONE', *, *, #2253, .F. ) ;
#8777=CARTESIAN_POINT ( 'NONE',  ( 2.624999999999998668, -28.77083333265053611, -4.546633369868303021 ) ) ;
#8782=CARTESIAN_POINT ( 'NONE',  ( -2.625000000000000444, -28.47916666598386826, -4.546633369868303021 ) ) ;
#8783=CARTESIAN_POINT ( 'NONE',  ( -1.406733260263391960, -27.63616454900183328, 5.250000000000000000 ) ) ;
#8787=CARTESIAN_POINT ( 'NONE',  ( 5.385316468750000141, -27.70312499965860198, -6.595110575850215044E-16 ) ) ;
#8791=CARTESIAN_POINT ( 'NONE',  ( 5.385316468750001029, -28.47395833299193413, 3.109213912904135846 ) ) ;
#8796=VERTEX_POINT ( 'NONE', #381 ) ;
#8803=ORIENTED_EDGE ( 'NONE', *, *, #761, .F. ) ;
#8810=CARTESIAN_POINT ( 'NONE',  ( 2.624999999999998668, -27.83333333333333215, -4.546633369868303021 ) ) ;
#8811=CARTESIAN_POINT ( 'NONE',  ( 5.385316468750000141, -28.48437499965860198, -6.595110575850215044E-16 ) ) ;
#8814=CARTESIAN_POINT ( 'NONE',  ( -5.385316468750000141, -28.10937499965860198, 0.000000000000000000 ) ) ;
#8819=CARTESIAN_POINT ( 'NONE',  ( 5.385316468749999252, -28.46354166632526628, -3.109213912904139399 ) ) ;
#8826=CARTESIAN_POINT ( 'NONE',  ( 2.624999999999998668, -27.27083333265053611, -4.546633369868303021 ) ) ;
#8827=CARTESIAN_POINT ( 'NONE',  ( 1.975475456537005874E-15, -27.68749999999999289, 5.250000000000000000 ) ) ;
#8831=CARTESIAN_POINT ( 'NONE',  ( 5.385316468750000141, -28.45312499965860198, -6.595110575850215044E-16 ) ) ;
#8833=CARTESIAN_POINT ( 'NONE',  ( -5.250000000000000000, -28.50000000000000000, 0.000000000000000000 ) ) ;
#8835=CARTESIAN_POINT ( 'NONE',  ( -5.385316468749998364, -28.05729166632526983, 3.109213912904140287 ) ) ;
#8840=VERTEX_POINT ( 'NONE', #4620 ) ;
#8841=CARTESIAN_POINT ( 'NONE',  ( 2.625000000000002220, -27.66666666666666430, 4.546633369868302132 ) ) ;
#8843=EDGE_CURVE ( 'NONE', #2470, #4857, #6095, .T. ) ;
#8854=CARTESIAN_POINT ( 'NONE',  ( -2.692658234375000514, -29.40104166632526983, -4.663820869356205989 ) ) ;
#8856=CARTESIAN_POINT ( 'NONE',  ( -3.807688866302469071E-16, -29.42187499965860198, -6.218427825808274356 ) ) ;
#8858=CARTESIAN_POINT ( 'NONE',  ( -9.180150650966086169E-15, -28.43750000000000000, 5.250000000000000000 ) ) ;
#8860=CARTESIAN_POINT ( 'NONE',  ( 2.692658234374998738, -29.19270833299193413, -4.663820869356206877 ) ) ;
#8862=CARTESIAN_POINT ( 'NONE',  ( -2.692658234375000514, -27.61979166632526628, -4.663820869356205989 ) ) ;
#8867=DIRECTION ( 'NONE',  ( 0.000000000000000000, -1.000000000000000000, 0.000000000000000000 ) ) ;
#8870=VERTEX_POINT ( 'NONE', #4555 ) ;
#8872=CARTESIAN_POINT ( 'NONE',  ( 1.142306659890740623E-15, -29.26562499965860198, 6.218427825808274356 ) ) ;
#8875=CARTESIAN_POINT ( 'NONE',  ( -2.692658234374996518, -28.53645833299193413, 4.663820869356208654 ) ) ;
#8884=CARTESIAN_POINT ( 'NONE',  ( -5.250000000000000000, -27.25000000000000000, 0.000000000000000000 ) ) ;
#8895=VECTOR ( 'NONE', #2745, 1000.000000000000000 ) ;
#8897=CARTESIAN_POINT ( 'NONE',  ( 0.000000000000000000, -30.00000000000000000, 0.000000000000000000 ) ) ;
#8898=CARTESIAN_POINT ( 'NONE',  ( -2.692658234374996518, -28.81770833299193413, 4.663820869356208654 ) ) ;
#8899=CARTESIAN_POINT ( 'NONE',  ( -5.385316468750000141, -29.60937499965859843, 0.000000000000000000 ) ) ;
#8903=AXIS2_PLACEMENT_3D ( 'NONE', #4263, #3481, #6306 ) ;
#8906=CARTESIAN_POINT ( 'NONE',  ( -2.692658234374996518, -29.81770833299193413, 4.663820869356208654 ) ) ;
#8909=CARTESIAN_POINT ( 'NONE',  ( -3.807688866302469071E-16, -28.39062499965860553, -6.218427825808274356 ) ) ;
#8915=CYLINDRICAL_SURFACE ( 'NONE', #8230, 5.250000000000000000 ) ;
#8921=CARTESIAN_POINT ( 'NONE',  ( -5.249999999999999112, -28.02083333333333215, -3.031088913245534755 ) ) ;
#8922=CARTESIAN_POINT ( 'NONE',  ( 2.692658234375002735, -28.74479166632526628, 4.663820869356205101 ) ) ;
#8925=ORIENTED_EDGE ( 'NONE', *, *, #4489, .F. ) ;
#8930=CARTESIAN_POINT ( 'NONE',  ( 5.250000000000000000, -28.12500000000000000, -6.429395695523604153E-16 ) ) ;
#8941=ADVANCED_FACE ( 'NONE', ( #1717 ), #4372, .F. ) ;
#8943=CARTESIAN_POINT ( 'NONE',  ( -3.807688866302469071E-16, -28.17187499965860198, -6.218427825808274356 ) ) ;
#8946=CARTESIAN_POINT ( 'NONE',  ( 5.385316468749999252, -28.96354166632526983, -3.109213912904139399 ) ) ;
#8948=VERTEX_POINT ( 'NONE', #1574 ) ;
#8950=CARTESIAN_POINT ( 'NONE',  ( 5.249999999999999112, -28.35416666666666785, -3.031088913245536975 ) ) ;
#8952=CARTESIAN_POINT ( 'NONE',  ( -3.807688866302469071E-16, -29.42187499965860198, -6.218427825808274356 ) ) ;
#8955=ORIENTED_EDGE ( 'NONE', *, *, #313, .F. ) ;
#8956=CARTESIAN_POINT ( 'NONE',  ( -5.385316468750000141, -28.07812499965860198, 0.000000000000000000 ) ) ;
#8959=EDGE_CURVE ( 'NONE', #6175, #2431, #7651, .T. ) ;
#8962=CARTESIAN_POINT ( 'NONE',  ( -2.624999999999996891, -28.39583333265053611, 4.546633369868304797 ) ) ;
#8967=CARTESIAN_POINT ( 'NONE',  ( 2.692658234375002735, -28.99479166632526983, 4.663820869356205101 ) ) ;
#8970=CARTESIAN_POINT ( 'NONE',  ( 5.385316468750000141, -29.20312499965859843, -6.595110575850215044E-16 ) ) ;
#8972=ORIENTED_EDGE ( 'NONE', *, *, #6696, .T. ) ;
#8979=CARTESIAN_POINT ( 'NONE',  ( -5.250000000000000000, -28.52083333333333215, -3.031088913245534755 ) ) ;
#8985=CARTESIAN_POINT ( 'NONE',  ( 6.429395695523604153E-16, -27.00000000000000000, 5.250000000000000000 ) ) ;
#8990=CARTESIAN_POINT ( 'NONE',  ( -5.385316468749998364, -28.83854166632527338, 3.109213912904140287 ) ) ;
#8993=CARTESIAN_POINT ( 'NONE',  ( -5.385316468750000141, -28.85937499965860198, 0.000000000000000000 ) ) ;
#8999=( BOUNDED_CURVE ( )  B_SPLINE_CURVE ( 2, ( #5810, #6291, #2772, #9083, #8648, #8352, #6330, #4807, #2280 ),
 .UNSPECIFIED., .F., .F. ) 
 B_SPLINE_CURVE_WITH_KNOTS ( ( 3, 2, 2, 2, 3 ),
 ( 0.5625000000000000000, 0.5694444444444444198, 0.5833333333333333703, 0.5972222222222222099, 0.6041666666666667407 ),
 .UNSPECIFIED. ) 
 CURVE ( )  GEOMETRIC_REPRESENTATION_ITEM ( )  RATIONAL_B_SPLINE_CURVE ( ( 0.9330127018922194093, 0.9330127018922194093, 1.000000000000000000, 0.8660254037844387076, 1.000000000000000000, 0.8660254037844387076, 1.000000000000000000, 0.9330127018922187432, 0.9330127018922192983 ) ) 
 REPRESENTATION_ITEM ( '' )  );
#9000=CARTESIAN_POINT ( 'NONE',  ( -5.385316468750000141, -29.85937499965859843, 0.000000000000000000 ) ) ;
#9001=EDGE_CURVE ( 'NONE', #7379, #3780, #7048, .T. ) ;
#9003=CARTESIAN_POINT ( 'NONE',  ( 5.385316468750000141, -28.45312499965860198, -6.595110575850215044E-16 ) ) ;
#9008=CYLINDRICAL_SURFACE ( 'NONE', #2430, 5.250000000000000000 ) ;
#9014=CARTESIAN_POINT ( 'NONE',  ( -3.807688866302469071E-16, -28.89062499965860198, -6.218427825808274356 ) ) ;
#9016=CARTESIAN_POINT ( 'NONE',  ( -9.180150650966086169E-15, -28.62499999931720396, 5.250000000000000000 ) ) ;
#9017=CARTESIAN_POINT ( 'NONE',  ( 2.692658234374998738, -29.66145833299193413, -4.663820869356206877 ) ) ;
#9024=ORIENTED_EDGE ( 'NONE', *, *, #5379, .F. ) ;
#9025=CARTESIAN_POINT ( 'NONE',  ( 5.250000000000000000, -28.10416666666666430, -3.031088913245536531 ) ) ;
#9030=PRODUCT_DEFINITION_FORMATION_WITH_SPECIFIED_SOURCE ( 'ANY', '', #5066, .NOT_KNOWN. ) ;
#9038=CARTESIAN_POINT ( 'NONE',  ( 5.250000000000000000, -29.31249999931720041, -6.429395695523604153E-16 ) ) ;
#9039=CARTESIAN_POINT ( 'NONE',  ( 5.385316468750001029, -30.00520833299193768, 3.109213912904134958 ) ) ;
#9041=CARTESIAN_POINT ( 'NONE',  ( -5.385316468750001029, -29.38020833299193413, -3.109213912904136734 ) ) ;
#9045=CARTESIAN_POINT ( 'NONE',  ( 5.250000000000000888, -28.39583333333333215, 3.031088913245533423 ) ) ;
#9047=CARTESIAN_POINT ( 'NONE',  ( 5.385316468749999252, -29.21354166632526628, -3.109213912904139399 ) ) ;
#9050=CARTESIAN_POINT ( 'NONE',  ( 5.385316468750000141, -27.95312499965860198, -6.595110575850215044E-16 ) ) ;
#9059=CARTESIAN_POINT ( 'NONE',  ( 1.045839947578414884E-14, -28.24999999931720041, -5.250000000000000000 ) ) ;
#9060=CONICAL_SURFACE ( 'NONE', #5199, 6.250000000000002665, 0.1221730476396033355 ) ;
#9062=CARTESIAN_POINT ( 'NONE',  ( 1.142306659890740623E-15, -29.51562499965859487, 6.218427825808274356 ) ) ;
#9065=CARTESIAN_POINT ( 'NONE',  ( 2.624999999999998668, -28.52083333265053611, -4.546633369868303021 ) ) ;
#9066=CARTESIAN_POINT ( 'NONE',  ( 2.692658234375002735, -29.24479166632526983, 4.663820869356205101 ) ) ;
#9072=CARTESIAN_POINT ( 'NONE',  ( -5.250000000000000000, -28.75000000000000000, 0.000000000000000000 ) ) ;
#9074=CIRCLE ( 'NONE', #8903, 2.786798956483056422 ) ;
#9078=CARTESIAN_POINT ( 'NONE',  ( -2.033577675846918216E-14, -29.93750000000000355, 5.250000000000000888 ) ) ;
#9081=DIRECTION ( 'NONE',  ( 0.000000000000000000, 0.000000000000000000, 1.000000000000000000 ) ) ;
#9083=CARTESIAN_POINT ( 'NONE',  ( -5.249999999999997335, -28.72916666666666785, 3.031088913245538308 ) ) ;
#9084=CARTESIAN_POINT ( 'NONE',  ( 2.624999999999998668, -29.27083333265053611, -4.546633369868303021 ) ) ;
#9091=CARTESIAN_POINT ( 'NONE',  ( -1.406733260263384411, -28.98883544963257464, -5.250000000000006217 ) ) ;
#9093=CARTESIAN_POINT ( 'NONE',  ( 1.142306659890740623E-15, -30.04687499965860198, 6.218427825808274356 ) ) ;
#9095=CARTESIAN_POINT ( 'NONE',  ( 5.385316468750001029, -29.47395833299193413, 3.109213912904134958 ) ) ;
#9100=DIRECTION ( 'NONE',  ( 0.000000000000000000, 0.000000000000000000, -1.000000000000000000 ) ) ;
#9101=CARTESIAN_POINT ( 'NONE',  ( 1.406733260263394847, -27.32366454968463287, -5.250000000000000000 ) ) ;
#9102=AXIS2_PLACEMENT_3D ( 'NONE', #9171, #4936, #4294 ) ;
#9104=CARTESIAN_POINT ( 'NONE',  ( 2.624999999999998668, -28.27083333265053255, -4.546633369868303021 ) ) ;
#9106=CARTESIAN_POINT ( 'NONE',  ( 5.250000000000000000, -27.81249999931720396, -6.429395695523604153E-16 ) ) ;
#9108=CARTESIAN_POINT ( 'NONE',  ( 1.975475456537005874E-15, -29.43750000000000000, 5.250000000000000000 ) ) ;
#9109=VECTOR ( 'NONE', #269, 1000.000000000000000 ) ;
#9110=CARTESIAN_POINT ( 'NONE',  ( -5.385316468750000141, -29.32812499965859843, 0.000000000000000000 ) ) ;
#9115=CARTESIAN_POINT ( 'NONE',  ( 6.429395695523604153E-16, -27.00000000000000000, 5.250000000000000000 ) ) ;
#9118=CARTESIAN_POINT ( 'NONE',  ( 5.250000000000000000, -29.60416666666666785, -3.031088913245536531 ) ) ;
#9122=DIRECTION ( 'NONE',  ( 0.000000000000000000, -1.000000000000000000, 0.000000000000000000 ) ) ;
#9128=CARTESIAN_POINT ( 'NONE',  ( -2.624999999999996891, -29.64583333265053611, 4.546633369868304797 ) ) ;
#9129=DIRECTION ( 'NONE',  ( 0.000000000000000000, -1.000000000000000000, 0.000000000000000000 ) ) ;
#9131=CARTESIAN_POINT ( 'NONE',  ( -5.317658234375000070, -30.03906249982930277, 0.000000000000000000 ) ) ;
#9136=CARTESIAN_POINT ( 'NONE',  ( 5.249999999999999112, -29.10416666666666785, -3.031088913245536975 ) ) ;
#9138=ORIENTED_EDGE ( 'NONE', *, *, #2917, .F. ) ;
#9139=CARTESIAN_POINT ( 'NONE',  ( -2.692658234374996518, -29.28645833299193413, 4.663820869356208654 ) ) ;
#9147=DIRECTION ( 'NONE',  ( 0.000000000000000000, -1.000000000000000000, 0.000000000000000000 ) ) ;
#9151=CARTESIAN_POINT ( 'NONE',  ( -5.385316468750000141, -27.10937499965860198, 0.000000000000000000 ) ) ;
#9156=CARTESIAN_POINT ( 'NONE',  ( -5.385316468750001029, -27.34895833299193768, -3.109213912904136734 ) ) ;
#9166=CARTESIAN_POINT ( 'NONE',  ( -5.249999999999999112, -29.27083333333333570, -3.031088913245534755 ) ) ;
#9167=CARTESIAN_POINT ( 'NONE',  ( -2.625000000000000444, -29.72916666598387181, -4.546633369868303021 ) ) ;
#9168=CARTESIAN_POINT ( 'NONE',  ( 1.406733260263395735, -27.61383544963257108, 5.250000000000000000 ) ) ;
#9169=EDGE_CURVE ( 'NONE', #8745, #2693, #5590, .T. ) ;
#9171=CARTESIAN_POINT ( 'NONE',  ( 0.000000000000000000, -27.00000000000000000, 0.000000000000000000 ) ) ;
#9175=CARTESIAN_POINT ( 'NONE',  ( 1.406733260263393293, -29.07366454968462577, -5.250000000000000000 ) ) ;
#9178=CARTESIAN_POINT ( 'NONE',  ( 5.385316468750000141, -29.95312499965859843, -6.595110575850215044E-16 ) ) ;
#9180=CARTESIAN_POINT ( 'NONE',  ( 6.429395695523604153E-16, -27.00000000000000000, 5.250000000000000000 ) ) ;
#9183=LINE ( 'NONE', #4908, #7893 ) ;
#9184=CARTESIAN_POINT ( 'NONE',  ( 0.000000000000000000, -27.00000000000000000, 0.000000000000000000 ) ) ;
#9185=CARTESIAN_POINT ( 'NONE',  ( 5.250000000000000000, -27.31249999931720396, -6.429395695523604153E-16 ) ) ;
#9233=COLOUR_RGB('Off White',0.89,0.88,0.83);
#9234=FILL_AREA_STYLE_COLOUR('',#9233);
#9235=FILL_AREA_STYLE('',(#9234));
#9236=SURFACE_STYLE_FILL_AREA(#9235);
#9237=SURFACE_SIDE_STYLE('',(#9236));
#9238=SURFACE_STYLE_USAGE(.BOTH.,#9237);
#9239=PRESENTATION_STYLE_ASSIGNMENT((#9238));
ENDSEC;
END-ISO-10303-21;
